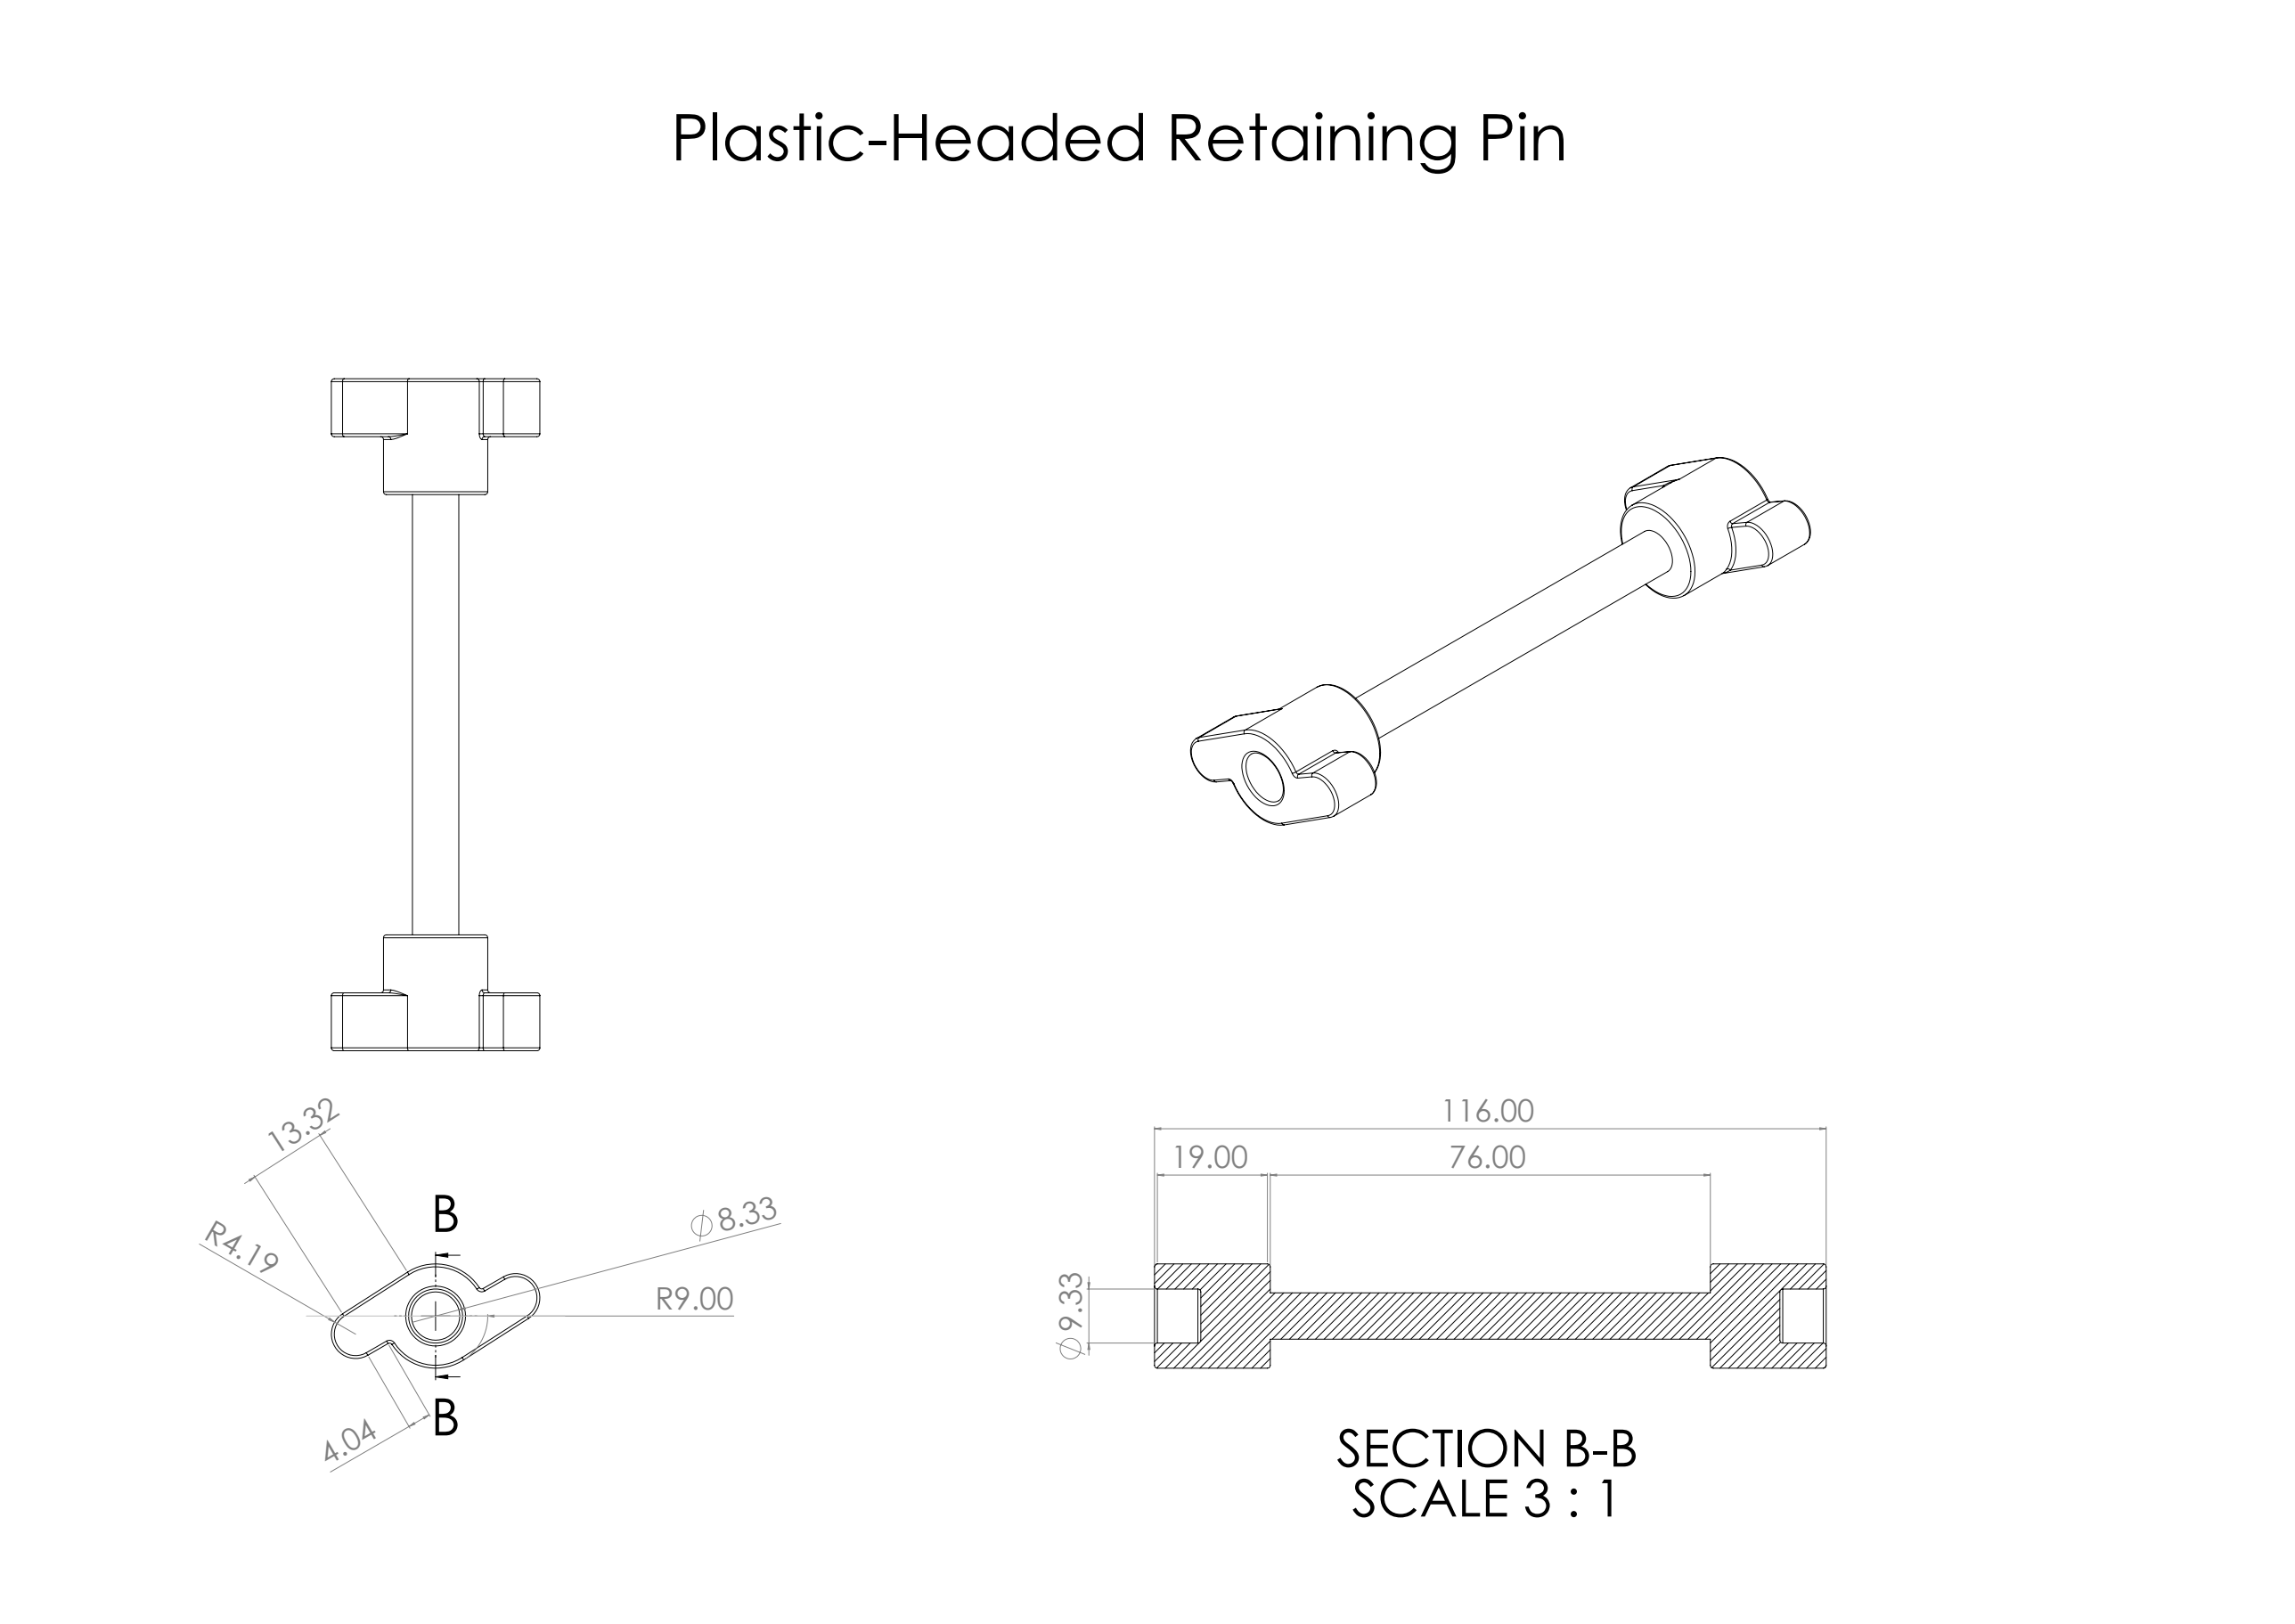
ISO-10303-21;
HEADER;
FILE_DESCRIPTION (('STEP AP214'),
    '1' );
FILE_NAME ('Plastic-Headed Retaining Pin.step',
    '2026-10-24T21:31:31',
    ( '' ),
    ( '' ),
    'SwSTEP 2.0',
    'SolidWorks 2025',
    '' );
FILE_SCHEMA (( 'AUTOMOTIVE_DESIGN' ));
ENDSEC;

DATA;
#1=AXIS2_PLACEMENT_3D ( 'NONE', #1022, #12813, #2258 ) ;
#8=EDGE_CURVE ( 'NONE', #12161, #11292, #4111, .T. ) ;
#15=ORIENTED_EDGE ( 'NONE', *, *, #6036, .T. ) ;
#28=FACE_OUTER_BOUND ( 'NONE', #3772, .T. ) ;
#31=CARTESIAN_POINT ( 'NONE',  ( -24.73111225919155132, -6.857688092579577344, -47.70917337021941762 ) ) ;
#34=ORIENTED_EDGE ( 'NONE', *, *, #2571, .T. ) ;
#45=CIRCLE ( 'NONE', #9384, 9.000000000000001776 ) ;
#48=CARTESIAN_POINT ( 'NONE',  ( -24.79038709231510040, -6.757381419356298657, 47.62582736825572738 ) ) ;
#51=ORIENTED_EDGE ( 'NONE', *, *, #11161, .F. ) ;
#53=VECTOR ( 'NONE', #9034, 1000.000000000000000 ) ;
#56=VERTEX_POINT ( 'NONE', #6360 ) ;
#60=VERTEX_POINT ( 'NONE', #14733 ) ;
#64=MECHANICAL_DESIGN_GEOMETRIC_PRESENTATION_REPRESENTATION('',(#7176),#14543);
#71=ORIENTED_EDGE ( 'NONE', *, *, #11240, .T. ) ;
#80=CIRCLE ( 'NONE', #11854, 0.5000000000000000000 ) ;
#83=CARTESIAN_POINT ( 'NONE',  ( -24.54250511040913096, 2.674312581063694516, -47.50000000000008527 ) ) ;
#90=DIRECTION ( 'NONE',  ( 0.000000000000000000, 0.000000000000000000, -1.000000000000000000 ) ) ;
#92=APPLICATION_CONTEXT ( 'automotive_design' ) ;
#93=CARTESIAN_POINT ( 'NONE',  ( -30.80945343098651890, -5.389243620311580329, -57.50000000000012079 ) ) ;
#103=( NAMED_UNIT ( * ) PLANE_ANGLE_UNIT ( ) SI_UNIT ( $, .RADIAN. ) );
#106=ORIENTED_EDGE ( 'NONE', *, *, #4616, .T. ) ;
#107=CARTESIAN_POINT ( 'NONE',  ( -9.038486528834313916, 1.949452350488303454, -47.50000000626571506 ) ) ;
#115=EDGE_LOOP ( 'NONE', ( #13949, #4522, #9265, #7527 ) ) ;
#119=CARTESIAN_POINT ( 'NONE',  ( -3.190546569013415379, 0.8906624217387615339, -57.50000000000012079 ) ) ;
#127=CARTESIAN_POINT ( 'NONE',  ( -25.21252699837112132, -6.998437922861948657, 48.50000000000011369 ) ) ;
#134=ORIENTED_EDGE ( 'NONE', *, *, #9339, .T. ) ;
#151=CARTESIAN_POINT ( 'NONE',  ( -22.13891797369473480, 5.141277655368648780, -48.38337049880507834 ) ) ;
#155=LINE ( 'NONE', #2612, #2752 ) ;
#160=DIRECTION ( 'NONE',  ( -0.000000000000000000, -0.000000000000000000, -1.000000000000000000 ) ) ;
#162=DIRECTION ( 'NONE',  ( 0.000000000000000000, 0.000000000000000000, 1.000000000000000000 ) ) ;
#164=CARTESIAN_POINT ( 'NONE',  ( -24.34296084301338681, 2.966536634491813818, 47.54128347412125066 ) ) ;
#165=EDGE_CURVE ( 'NONE', #11054, #3062, #11494, .T. ) ;
#169=AXIS2_PLACEMENT_3D ( 'NONE', #4841, #13010, #2308 ) ;
#170=VERTEX_POINT ( 'NONE', #13972 ) ;
#172=LINE ( 'NONE', #1320, #11742 ) ;
#175=CARTESIAN_POINT ( 'NONE',  ( -9.097850607046364502, 2.059891325575069043, -47.52616914649232172 ) ) ;
#193=TOROIDAL_SURFACE ( 'NONE', #8776, 5.165819364273509073, 0.5000000000000000000 ) ;
#198=CARTESIAN_POINT ( 'NONE',  ( -25.01741698508091005, -6.338425579613558014, 48.00000000000010658 ) ) ;
#202=ADVANCED_FACE ( 'NONE', ( #3509 ), #12825, .F. ) ;
#203=VECTOR ( 'NONE', #10665, 1000.000000000000000 ) ;
#210=CARTESIAN_POINT ( 'NONE',  ( 1.004339113574583608, 0.8906624217387615339, -48.00000000000012079 ) ) ;
#214=EDGE_CURVE ( 'NONE', #14442, #11277, #7315, .T. ) ;
#215=CIRCLE ( 'NONE', #445, 0.5000000000000000000 ) ;
#217=DIRECTION ( 'NONE',  ( -0.000000000000000000, 0.000000000000000000, 1.000000000000000000 ) ) ;
#219=DIRECTION ( 'NONE',  ( 0.8420378618367728718, 0.5394184268574404584, -0.000000000000000000 ) ) ;
#229=AXIS2_PLACEMENT_3D ( 'NONE', #14012, #3468, #10624 ) ;
#231=EDGE_LOOP ( 'NONE', ( #10918, #12061, #5408, #5048 ) ) ;
#241=CARTESIAN_POINT ( 'NONE',  ( -28.95977857253349796, -8.587818791446737876, 48.00000000000012079 ) ) ;
#244=CARTESIAN_POINT ( 'NONE',  ( -23.91311688008704905, 3.524160940036151324, 47.66502101098827637 ) ) ;
#250=CIRCLE ( 'NONE', #10335, 1.000000000000000888 ) ;
#253=CARTESIAN_POINT ( 'NONE',  ( -10.99067925302910176, -8.982598353005794678, -48.14374739243442747 ) ) ;
#267=FACE_OUTER_BOUND ( 'NONE', #14593, .T. ) ;
#269=ORIENTED_EDGE ( 'NONE', *, *, #14642, .F. ) ;
#274=CARTESIAN_POINT ( 'NONE',  ( -24.96483633670257873, -6.441926561070030033, 48.01692658285762150 ) ) ;
#282=AXIS2_PLACEMENT_3D ( 'NONE', #9055, #1887, #6818 ) ;
#284=EDGE_CURVE ( 'NONE', #12776, #11451, #5880, .T. ) ;
#290=CARTESIAN_POINT ( 'NONE',  ( -25.46282903980762669, -6.565599745187292946, 47.50000000000012079 ) ) ;
#296=ORIENTED_EDGE ( 'NONE', *, *, #1661, .T. ) ;
#298=VERTEX_POINT ( 'NONE', #5547 ) ;
#303=FACE_OUTER_BOUND ( 'NONE', #6423, .T. ) ;
#310=CIRCLE ( 'NONE', #8176, 4.665819364273509073 ) ;
#319=FACE_OUTER_BOUND ( 'NONE', #4555, .T. ) ;
#324=ORIENTED_EDGE ( 'NONE', *, *, #7653, .T. ) ;
#329=CARTESIAN_POINT ( 'NONE',  ( -9.191242442328487527, 2.249476921181321476, -48.36238429206942868 ) ) ;
#336=CIRCLE ( 'NONE', #6243, 3.694885682587998765 ) ;
#342=DIRECTION ( 'NONE',  ( 0.000000000000000000, 0.000000000000000000, 1.000000000000000000 ) ) ;
#345=DIRECTION ( 'NONE',  ( 0.000000000000000000, -0.000000000000000000, -1.000000000000000000 ) ) ;
#349=EDGE_CURVE ( 'NONE', #13079, #8396, #2395, .T. ) ;
#350=DIRECTION ( 'NONE',  ( -0.8656763553493062036, -0.5006040828730242698, -0.000000000000000000 ) ) ;
#353=ORIENTED_EDGE ( 'NONE', *, *, #9943, .F. ) ;
#355=VERTEX_POINT ( 'NONE', #12871 ) ;
#356=CARTESIAN_POINT ( 'NONE',  ( -25.46282903980762669, -6.565599745187292946, 48.00000000000012079 ) ) ;
#361=CARTESIAN_POINT ( 'NONE',  ( -32.80254285330622110, -2.278009980413880697, -48.50000000000012079 ) ) ;
#372=DIRECTION ( 'NONE',  ( 1.000000000000000000, 0.000000000000000000, 0.000000000000000000 ) ) ;
#373=ORIENTED_EDGE ( 'NONE', *, *, #13891, .T. ) ;
#375=ORIENTED_EDGE ( 'NONE', *, *, #2546, .T. ) ;
#376=DIRECTION ( 'NONE',  ( -0.000000000000000000, -0.000000000000000000, -1.000000000000000000 ) ) ;
#385=CARTESIAN_POINT ( 'NONE',  ( -24.57377864815406099, 2.621914368698142983, 47.92899112040971943 ) ) ;
#386=EDGE_CURVE ( 'NONE', #5046, #7147, #1076, .T. ) ;
#388=EDGE_CURVE ( 'NONE', #5785, #8918, #8303, .T. ) ;
#396=CARTESIAN_POINT ( 'NONE',  ( -10.31873516982594907, -8.289185193041582522, -47.74939190649462972 ) ) ;
#397=AXIS2_PLACEMENT_3D ( 'NONE', #6924, #8082, #15007 ) ;
#403=CARTESIAN_POINT ( 'NONE',  ( -8.729485970062036415, 2.417371407811747197, 48.19241902544784750 ) ) ;
#413=AXIS2_PLACEMENT_3D ( 'NONE', #11900, #10826, #1359 ) ;
#415=CARTESIAN_POINT ( 'NONE',  ( -25.21252699939434194, -6.998437923453657561, -48.43453164808065736 ) ) ;
#419=ADVANCED_BREP_SHAPE_REPRESENTATION ( '', ( #14292, #6315 ), #9517 ) ;
#426=AXIS2_PLACEMENT_3D ( 'NONE', #9506, #14202, #3798 ) ;
#429=DIRECTION ( 'NONE',  ( 0.000000000000000000, 0.000000000000000000, 1.000000000000000000 ) ) ;
#434=ORIENTED_EDGE ( 'NONE', *, *, #386, .T. ) ;
#443=ORIENTED_EDGE ( 'NONE', *, *, #5395, .T. ) ;
#444=CARTESIAN_POINT ( 'NONE',  ( -23.91237149244958360, 3.525053131390499139, 47.66527511103321046 ) ) ;
#445=AXIS2_PLACEMENT_3D ( 'NONE', #12775, #5776, #7923 ) ;
#451=AXIS2_PLACEMENT_3D ( 'NONE', #9024, #9337, #11476 ) ;
#452=CARTESIAN_POINT ( 'NONE',  ( -24.54316048551696028, -7.158540021523408292, 58.00000000000012079 ) ) ;
#455=DIRECTION ( 'NONE',  ( -0.5394184268574523378, 0.8420378618367652113, 0.000000000000000000 ) ) ;
#458=LINE ( 'NONE', #7761, #5187 ) ;
#459=DIRECTION ( 'NONE',  ( -0.5394184268574406804, 0.8420378618367728718, 0.000000000000000000 ) ) ;
#469=CARTESIAN_POINT ( 'NONE',  ( -9.657716696386627220, -7.466071317230740689, -47.54143911729025973 ) ) ;
#473=DIRECTION ( 'NONE',  ( -0.8420378618367644341, -0.5394184268574535590, -0.000000000000000000 ) ) ;
#478=CARTESIAN_POINT ( 'NONE',  ( -9.107478285483566083, 2.086796655788927701, 48.09696226170978406 ) ) ;
#485=EDGE_CURVE ( 'NONE', #14513, #11292, #5381, .T. ) ;
#486=AXIS2_PLACEMENT_3D ( 'NONE', #549, #8705, #618 ) ;
#487=EDGE_CURVE ( 'NONE', #14705, #9017, #2919, .T. ) ;
#490=VERTEX_POINT ( 'NONE', #4780 ) ;
#492=ORIENTED_EDGE ( 'NONE', *, *, #7012, .F. ) ;
#493=CARTESIAN_POINT ( 'NONE',  ( -25.24562193491511763, -6.954963132161501527, 48.23869654929341522 ) ) ;
#495=VECTOR ( 'NONE', #4431, 1000.000000000000000 ) ;
#498=ORIENTED_EDGE ( 'NONE', *, *, #9078, .F. ) ;
#499=PLANE ( 'NONE',  #14653 ) ;
#503=EDGE_CURVE ( 'NONE', #4611, #7961, #14234, .T. ) ;
#505=VERTEX_POINT ( 'NONE', #2771 ) ;
#509=ORIENTED_EDGE ( 'NONE', *, *, #3414, .F. ) ;
#511=ORIENTED_EDGE ( 'NONE', *, *, #11557, .T. ) ;
#516=DIRECTION ( 'NONE',  ( 0.000000000000000000, 0.000000000000000000, -1.000000000000000000 ) ) ;
#522=CIRCLE ( 'NONE', #13552, 0.5000000000000004441 ) ;
#528=DIRECTION ( 'NONE',  ( 1.000000000000000000, 0.000000000000000000, 0.000000000000000000 ) ) ;
#532=VECTOR ( 'NONE', #9239, 1000.000000000000000 ) ;
#545=AXIS2_PLACEMENT_3D ( 'NONE', #1167, #6104, #8339 ) ;
#546=ORIENTED_EDGE ( 'NONE', *, *, #487, .F. ) ;
#548=CIRCLE ( 'NONE', #9166, 0.5000000000000000000 ) ;
#549=CARTESIAN_POINT ( 'NONE',  ( -3.190546569013415379, 0.8906624217387615339, 48.50000000000012079 ) ) ;
#593=CARTESIAN_POINT ( 'NONE',  ( -9.657716696386627220, -7.466071317230740689, 47.54143911729025973 ) ) ;
#594=ORIENTED_EDGE ( 'NONE', *, *, #11102, .F. ) ;
#601=EDGE_LOOP ( 'NONE', ( #14385, #13165, #13920, #13167 ) ) ;
#603=ORIENTED_EDGE ( 'NONE', *, *, #12571, .F. ) ;
#616=ORIENTED_EDGE ( 'NONE', *, *, #4933, .T. ) ;
#618=DIRECTION ( 'NONE',  ( 1.000000000000000000, 0.000000000000000000, 0.000000000000000000 ) ) ;
#631=ORIENTED_EDGE ( 'NONE', *, *, #11253, .F. ) ;
#636=ORIENTED_EDGE ( 'NONE', *, *, #8900, .T. ) ;
#641=EDGE_CURVE ( 'NONE', #13513, #7657, #11510, .T. ) ;
#646=AXIS2_PLACEMENT_3D ( 'NONE', #2800, #14494, #8783 ) ;
#655=DIRECTION ( 'NONE',  ( 1.000000000000000000, 0.000000000000000000, 0.000000000000000000 ) ) ;
#663=EDGE_CURVE ( 'NONE', #4371, #14705, #1159, .T. ) ;
#664=DIRECTION ( 'NONE',  ( 1.000000000000000000, 0.000000000000000000, 0.000000000000000000 ) ) ;
#670=CARTESIAN_POINT ( 'NONE',  ( -32.80254285330626374, -2.278009980413908231, 48.50000000000012079 ) ) ;
#673=FACE_OUTER_BOUND ( 'NONE', #12478, .T. ) ;
#674=ORIENTED_EDGE ( 'NONE', *, *, #4052, .T. ) ;
#677=ORIENTED_EDGE ( 'NONE', *, *, #11895, .F. ) ;
#681=CARTESIAN_POINT ( 'NONE',  ( -24.66543232906180805, 3.122884019241207287, -48.02064173568555816 ) ) ;
#683=ORIENTED_EDGE ( 'NONE', *, *, #5858, .F. ) ;
#687=CARTESIAN_POINT ( 'NONE',  ( 0.000000000000000000, 0.000000000000000000, -38.00000000000012079 ) ) ;
#693=CARTESIAN_POINT ( 'NONE',  ( -16.99999999999998579, -2.249290599286303927, -57.50000000000012079 ) ) ;
#705=CARTESIAN_POINT ( 'NONE',  ( -24.55671735758753726, -7.137878559097176279, -48.23807154671105479 ) ) ;
#707=EDGE_CURVE ( 'NONE', #355, #7994, #45, .T. ) ;
#718=AXIS2_PLACEMENT_3D ( 'NONE', #2213, #10452, #821 ) ;
#727=EDGE_LOOP ( 'NONE', ( #10150, #492, #10188, #14509 ) ) ;
#730=FACE_OUTER_BOUND ( 'NONE', #5305, .T. ) ;
#744=CYLINDRICAL_SURFACE ( 'NONE', #11640, 0.4999999999999996669 ) ;
#746=AXIS2_PLACEMENT_3D ( 'NONE', #2112, #5754, #6809 ) ;
#748=DIRECTION ( 'NONE',  ( 0.5006040828730401460, -0.8656763553492970997, 0.000000000000000000 ) ) ;
#752=CARTESIAN_POINT ( 'NONE',  ( -21.58505662828840599, 4.908031226326156293, -57.50000000000012079 ) ) ;
#754=CIRCLE ( 'NONE', #12822, 0.4999999999999997224 ) ;
#763=LINE ( 'NONE', #1921, #4404 ) ;
#769=TOROIDAL_SURFACE ( 'NONE', #2002, 3.694885682587998765, 0.5000000000000000000 ) ;
#776=DIRECTION ( 'NONE',  ( 0.000000000000000000, 0.000000000000000000, -1.000000000000000000 ) ) ;
#779=AXIS2_PLACEMENT_3D ( 'NONE', #15041, #4571, #14877 ) ;
#781=AXIS2_PLACEMENT_3D ( 'NONE', #13323, #5092, #9797 ) ;
#785=CARTESIAN_POINT ( 'NONE',  ( -8.499999999999987566, -2.249290599286303927, -38.00000000000012079 ) ) ;
#789=CYLINDRICAL_SURFACE ( 'NONE', #12032, 4.194885682588113340 ) ;
#805=DIRECTION ( 'NONE',  ( 1.000000000000000000, 0.000000000000000000, 0.000000000000000000 ) ) ;
#821=DIRECTION ( 'NONE',  ( 1.000000000000000000, 0.000000000000000000, 0.000000000000000000 ) ) ;
#825=ORIENTED_EDGE ( 'NONE', *, *, #1492, .T. ) ;
#842=DIRECTION ( 'NONE',  ( -0.000000000000000000, -0.000000000000000000, -1.000000000000000000 ) ) ;
#851=ADVANCED_FACE ( 'NONE', ( #9652 ), #14341, .F. ) ;
#856=DIRECTION ( 'NONE',  ( 0.000000000000000000, -1.000000000000000000, 0.000000000000000000 ) ) ;
#859=FACE_OUTER_BOUND ( 'NONE', #13100, .T. ) ;
#864=VERTEX_POINT ( 'NONE', #12532 ) ;
#872=DIRECTION ( 'NONE',  ( 0.000000000000000000, 0.000000000000000000, -1.000000000000000000 ) ) ;
#877=DIRECTION ( 'NONE',  ( 1.000000000000000000, 0.000000000000000000, 0.000000000000000000 ) ) ;
#887=CARTESIAN_POINT ( 'NONE',  ( -16.99999999999998579, -2.249290599286303927, -58.00000000000012079 ) ) ;
#888=CIRCLE ( 'NONE', #9509, 0.4999999999999997780 ) ;
#890=CARTESIAN_POINT ( 'NONE',  ( -8.537170960192302260, 2.067018546614596719, -48.00000000000012079 ) ) ;
#892=AXIS2_PLACEMENT_3D ( 'NONE', #6524, #1690, #528 ) ;
#894=ORIENTED_EDGE ( 'NONE', *, *, #4866, .T. ) ;
#896=DIRECTION ( 'NONE',  ( 1.000000000000000000, 0.000000000000000000, 0.000000000000000000 ) ) ;
#901=EDGE_CURVE ( 'NONE', #298, #3805, #11869, .T. ) ;
#903=CARTESIAN_POINT ( 'NONE',  ( -7.499999999999985789, -2.249290599286303927, 47.50000000000012079 ) ) ;
#904=VECTOR ( 'NONE', #10762, 1000.000000000000114 ) ;
#912=CARTESIAN_POINT ( 'NONE',  ( -21.85476584171706449, 5.329050157244580532, -48.50000000000012079 ) ) ;
#915=EDGE_LOOP ( 'NONE', ( #9268, #4270, #12205, #3537 ) ) ;
#922=VERTEX_POINT ( 'NONE', #11287 ) ;
#933=CARTESIAN_POINT ( 'NONE',  ( -8.787473000605775297, 2.499856724880853864, -48.43453164808066447 ) ) ;
#934=CARTESIAN_POINT ( 'NONE',  ( -33.07225206673494711, -1.856991049495498425, -48.50000000000012079 ) ) ;
#936=DIRECTION ( 'NONE',  ( 0.8420378618367728718, 0.5394184268574404584, 0.000000000000000000 ) ) ;
#944=CARTESIAN_POINT ( 'NONE',  ( -28.70947653109703523, -9.020656969121422009, -57.50000000000012079 ) ) ;
#952=AXIS2_PLACEMENT_3D ( 'NONE', #10166, #3233, #14775 ) ;
#953=( BOUNDED_SURFACE ( )  B_SPLINE_SURFACE ( 3, 2, ( 
 ( #11003, #4136, #12769 ),
 ( #2218, #2299, #5613 ),
 ( #975, #5847, #11363 ),
 ( #7840, #12685, #2137 ),
 ( #3216, #9227, #15146 ),
 ( #15078, #3141, #6830 ),
 ( #14908, #3450, #10455 ),
 ( #8147, #10379, #10303 ) ),
 .UNSPECIFIED., .F., .F., .F. ) 
 B_SPLINE_SURFACE_WITH_KNOTS ( ( 4, 2, 2, 4 ),
 ( 3, 3 ),
 ( -6.505213034913026604E-19, 0.001129222206655588513, 0.002258444413311177894, 0.004516888826622356655 ),
 ( 0.000000000000000000, 1.000000000000000000 ),
 .UNSPECIFIED. ) 
 GEOMETRIC_REPRESENTATION_ITEM ( )  RATIONAL_B_SPLINE_SURFACE ( (
 ( 1.000000000000000000, 0.7071067811864926167, 1.000000000000000000),
 ( 1.000000000000000000, 0.7608707698419998611, 1.000000000000000000),
 ( 1.000000000000000000, 0.8047257278452493168, 1.000000000000000000),
 ( 1.000000000000000000, 0.8783509392183369568, 1.000000000000000000),
 ( 1.000000000000000000, 0.9081758943107525184, 1.000000000000000000),
 ( 1.000000000000000000, 0.9781389570701306546, 1.000000000000000000),
 ( 1.000000000000000000, 0.9996704379322433054, 1.000000000000000000),
 ( 1.000000000000000000, 1.000000000000000000, 1.000000000000000000) ) ) 
 REPRESENTATION_ITEM ( '' )  SURFACE ( )  );
#954=DIRECTION ( 'NONE',  ( 0.8420378618367644341, 0.5394184268574535590, 0.000000000000000000 ) ) ;
#956=CARTESIAN_POINT ( 'NONE',  ( 0.6601805061683232445, -1.030548743169294346, 57.50000000000012079 ) ) ;
#961=ORIENTED_EDGE ( 'NONE', *, *, #6671, .T. ) ;
#964=AXIS2_PLACEMENT_3D ( 'NONE', #11793, #936, #4486 ) ;
#968=ORIENTED_EDGE ( 'NONE', *, *, #5858, .T. ) ;
#971=FACE_OUTER_BOUND ( 'NONE', #5210, .T. ) ;
#974=EDGE_CURVE ( 'NONE', #11391, #10817, #14814, .T. ) ;
#975=CARTESIAN_POINT ( 'NONE',  ( -9.657039156986668260, -7.465117833064532249, 47.54128347411995037 ) ) ;
#981=VERTEX_POINT ( 'NONE', #6749 ) ;
#986=CYLINDRICAL_SURFACE ( 'NONE', #5207, 4.665819364273509073 ) ;
#988=ORIENTED_EDGE ( 'NONE', *, *, #12071, .F. ) ;
#990=VECTOR ( 'NONE', #350, 1000.000000000000000 ) ;
#994=DIRECTION ( 'NONE',  ( -0.000000000000000000, -0.000000000000000000, -1.000000000000000000 ) ) ;
#1006=ORIENTED_EDGE ( 'NONE', *, *, #15185, .F. ) ;
#1009=EDGE_LOOP ( 'NONE', ( #9822, #6669, #1334, #10838 ) ) ;
#1014=PLANE ( 'NONE',  #7092 ) ;
#1021=ORIENTED_EDGE ( 'NONE', *, *, #8257, .F. ) ;
#1022=CARTESIAN_POINT ( 'NONE',  ( -24.96222495693456978, -7.431276100536581275, -48.50000000000012079 ) ) ;
#1028=PLANE ( 'NONE',  #14565 ) ;
#1031=EDGE_CURVE ( 'NONE', #922, #3003, #2788, .T. ) ;
#1048=LINE ( 'NONE', #210, #4481 ) ;
#1050=CARTESIAN_POINT ( 'NONE',  ( 1.004339113574583608, 0.8906624217387615339, 48.00000000000012079 ) ) ;
#1055=AXIS2_PLACEMENT_3D ( 'NONE', #3787, #9729, #7919 ) ;
#1057=VECTOR ( 'NONE', #994, 1000.000000000000000 ) ;
#1069=VECTOR ( 'NONE', #4442, 1000.000000000000000 ) ;
#1070=EDGE_LOOP ( 'NONE', ( #1164, #3149 ) ) ;
#1076=LINE ( 'NONE', #3311, #11234 ) ;
#1081=DIRECTION ( 'NONE',  ( -0.000000000000000000, -0.000000000000000000, -1.000000000000000000 ) ) ;
#1097=ADVANCED_FACE ( 'NONE', ( #8307 ), #11826, .F. ) ;
#1106=DIRECTION ( 'NONE',  ( -0.000000000000000000, 1.000000000000000000, 0.000000000000000000 ) ) ;
#1108=DIRECTION ( 'NONE',  ( 1.000000000000000000, 0.000000000000000000, 0.000000000000000000 ) ) ;
#1122=DIRECTION ( 'NONE',  ( 1.000000000000000000, 0.000000000000000000, 0.000000000000000000 ) ) ;
#1124=EDGE_CURVE ( 'NONE', #11720, #12161, #8919, .T. ) ;
#1125=VERTEX_POINT ( 'NONE', #10604 ) ;
#1133=VECTOR ( 'NONE', #7599, 1000.000000000000000 ) ;
#1142=ORIENTED_EDGE ( 'NONE', *, *, #4718, .F. ) ;
#1152=AXIS2_PLACEMENT_3D ( 'NONE', #12756, #4427, #9132 ) ;
#1159=CIRCLE ( 'NONE', #5842, 0.5000000000000008882 ) ;
#1164=ORIENTED_EDGE ( 'NONE', *, *, #7456, .T. ) ;
#1167=CARTESIAN_POINT ( 'NONE',  ( -32.80254285330622110, -2.278009980413880697, 48.50000000000012079 ) ) ;
#1170=CIRCLE ( 'NONE', #6821, 9.500000000000001776 ) ;
#1172=FACE_OUTER_BOUND ( 'NONE', #2030, .T. ) ;
#1174=AXIS2_PLACEMENT_3D ( 'NONE', #11340, #12661, #954 ) ;
#1187=CARTESIAN_POINT ( 'NONE',  ( -8.842479278987921631, -7.118053859731281463, -48.00000000000012079 ) ) ;
#1197=CARTESIAN_POINT ( 'NONE',  ( -16.99999999999998579, -2.249290599286303927, 50.00000000000012079 ) ) ;
#1198=CARTESIAN_POINT ( 'NONE',  ( -25.46282903980763024, -6.565599745187293834, 48.00000000000012079 ) ) ;
#1204=DIRECTION ( 'NONE',  ( 0.5454721580263366398, -0.8381289428352246551, 4.385647630081457888E-16 ) ) ;
#1220=EDGE_LOOP ( 'NONE', ( #9030, #9222, #106, #3497 ) ) ;
#1223=CARTESIAN_POINT ( 'NONE',  ( -23.91237149244958360, 3.525053131390499139, -47.66527511103321046 ) ) ;
#1228=FACE_OUTER_BOUND ( 'NONE', #1806, .T. ) ;
#1238=ORIENTED_EDGE ( 'NONE', *, *, #9123, .F. ) ;
#1244=DIRECTION ( 'NONE',  ( 0.000000000000000000, 0.000000000000000000, 1.000000000000000000 ) ) ;
#1248=PLANE ( 'NONE',  #2409 ) ;
#1252=AXIS2_PLACEMENT_3D ( 'NONE', #11270, #13666, #13822 ) ;
#1253=EDGE_LOOP ( 'NONE', ( #1021, #5256, #6232, #324 ) ) ;
#1259=FACE_OUTER_BOUND ( 'NONE', #10043, .T. ) ;
#1268=CARTESIAN_POINT ( 'NONE',  ( -25.43628086306388525, -6.625164433253370788, 48.00000000000012079 ) ) ;
#1273=AXIS2_PLACEMENT_3D ( 'NONE', #8800, #13496, #6352 ) ;
#1282=AXIS2_PLACEMENT_3D ( 'NONE', #2665, #5347, #6422 ) ;
#1291=DIRECTION ( 'NONE',  ( 0.000000000000000000, 0.000000000000000000, -1.000000000000000000 ) ) ;
#1295=FACE_OUTER_BOUND ( 'NONE', #8669, .T. ) ;
#1304=CARTESIAN_POINT ( 'NONE',  ( -24.12409601409935078, -6.885803942510236197, -57.50000000000012079 ) ) ;
#1307=CARTESIAN_POINT ( 'NONE',  ( -30.80945343098651890, -5.389243620311580329, -48.00000000000012079 ) ) ;
#1309=EDGE_CURVE ( 'NONE', #12008, #14442, #8458, .T. ) ;
#1310=DIRECTION ( 'NONE',  ( -0.8656763553492639041, -0.5006040828730973224, 0.000000000000000000 ) ) ;
#1317=CARTESIAN_POINT ( 'NONE',  ( -3.190546569013415379, 0.8906624217387615339, 48.50000000000012079 ) ) ;
#1320=CARTESIAN_POINT ( 'NONE',  ( -28.70947653109703168, -9.020656969121420232, 48.00000000000012079 ) ) ;
#1326=EDGE_CURVE ( 'NONE', #7147, #298, #13221, .T. ) ;
#1328=EDGE_CURVE ( 'NONE', #505, #1125, #2947, .T. ) ;
#1334=ORIENTED_EDGE ( 'NONE', *, *, #12288, .T. ) ;
#1335=EDGE_CURVE ( 'NONE', #6376, #5507, #5755, .T. ) ;
#1337=FACE_OUTER_BOUND ( 'NONE', #5812, .T. ) ;
#1340=DIRECTION ( 'NONE',  ( 1.000000000000000000, 0.000000000000000000, 0.000000000000000000 ) ) ;
#1343=CARTESIAN_POINT ( 'NONE',  ( -8.537170960192327129, 2.067018546614582508, 57.50000000000012079 ) ) ;
#1353=PRODUCT_DEFINITION_CONTEXT ( 'detailed design', #5158, 'design' ) ;
#1357=ORIENTED_EDGE ( 'NONE', *, *, #5945, .T. ) ;
#1359=DIRECTION ( 'NONE',  ( 1.000000000000000000, 0.000000000000000000, 0.000000000000000000 ) ) ;
#1366=LINE ( 'NONE', #2596, #12722 ) ;
#1368=ORIENTED_EDGE ( 'NONE', *, *, #8899, .T. ) ;
#1375=VERTEX_POINT ( 'NONE', #4186 ) ;
#1388=DIRECTION ( 'NONE',  ( -0.4543483311474630915, 0.8908241094534405935, -0.000000000000000000 ) ) ;
#1390=CARTESIAN_POINT ( 'NONE',  ( -24.54301448188264700, 2.673459138797629198, 47.50000001881890910 ) ) ;
#1393=CIRCLE ( 'NONE', #3357, 9.000000000000001776 ) ;
#1395=AXIS2_PLACEMENT_3D ( 'NONE', #2267, #15123, #11570 ) ;
#1399=CARTESIAN_POINT ( 'NONE',  ( -9.209612907684750382, 2.258800220783480750, -47.62582736825572738 ) ) ;
#1402=DIRECTION ( 'NONE',  ( 1.000000000000000000, 0.000000000000000000, 0.000000000000000000 ) ) ;
#1409=AXIS2_PLACEMENT_3D ( 'NONE', #11979, #4986, #10916 ) ;
#1421=CARTESIAN_POINT ( 'NONE',  ( -24.90214939295363550, -6.558472524147630267, 47.52616914649232172 ) ) ;
#1437=CIRCLE ( 'NONE', #6552, 0.5000000000000004441 ) ;
#1450=ORIENTED_EDGE ( 'NONE', *, *, #5868, .T. ) ;
#1453=ORIENTED_EDGE ( 'NONE', *, *, #4286, .F. ) ;
#1454=CARTESIAN_POINT ( 'NONE',  ( -16.99999999999998579, -2.249290599286303927, -47.50000000000012079 ) ) ;
#1455=CARTESIAN_POINT ( 'NONE',  ( -11.05444845021228595, -9.014367880605227867, 48.04486892757390848 ) ) ;
#1458=CARTESIAN_POINT ( 'NONE',  ( -3.285520523750506516, 5.681530634152946568, 48.00000000000012079 ) ) ;
#1462=( BOUNDED_SURFACE ( )  B_SPLINE_SURFACE ( 3, 2, ( 
 ( #5640, #10330, #9182 ),
 ( #13867, #8020, #12719 ),
 ( #5726, #9253, #13947 ),
 ( #8099, #12800, #14104 ),
 ( #2402, #10482, #11935 ),
 ( #11708, #253, #13104 ),
 ( #10566, #3556, #4711 ),
 ( #9573, #2479, #10713 ) ),
 .UNSPECIFIED., .F., .F., .F. ) 
 B_SPLINE_SURFACE_WITH_KNOTS ( ( 4, 2, 2, 4 ),
 ( 3, 3 ),
 ( -6.505213034913026604E-19, 0.001129222206655588513, 0.002258444413311177894, 0.004516888826622356655 ),
 ( 0.000000000000000000, 1.000000000000000000 ),
 .UNSPECIFIED. ) 
 GEOMETRIC_REPRESENTATION_ITEM ( )  RATIONAL_B_SPLINE_SURFACE ( (
 ( 1.000000000000000000, 0.7071067811864926167, 1.000000000000000000),
 ( 1.000000000000000000, 0.7608707698419998611, 1.000000000000000000),
 ( 1.000000000000000000, 0.8047257278452493168, 1.000000000000000000),
 ( 1.000000000000000000, 0.8783509392183369568, 1.000000000000000000),
 ( 1.000000000000000000, 0.9081758943107525184, 1.000000000000000000),
 ( 1.000000000000000000, 0.9781389570701306546, 1.000000000000000000),
 ( 1.000000000000000000, 0.9996704379322433054, 1.000000000000000000),
 ( 1.000000000000000000, 1.000000000000000000, 1.000000000000000000) ) ) 
 REPRESENTATION_ITEM ( '' )  SURFACE ( )  );
#1468=CARTESIAN_POINT ( 'NONE',  ( -0.9277479332649583021, -2.641590149077306826, -48.00000000000012079 ) ) ;
#1469=ORIENTED_EDGE ( 'NONE', *, *, #9614, .T. ) ;
#1473=AXIS2_PLACEMENT_3D ( 'NONE', #2874, #6349, #7729 ) ;
#1484=CARTESIAN_POINT ( 'NONE',  ( -25.01741698508091005, -6.338425579613558014, 47.50000000000012079 ) ) ;
#1485=CIRCLE ( 'NONE', #9354, 0.5000000000000001110 ) ;
#1488=CARTESIAN_POINT ( 'NONE',  ( -9.263396839842437558, 2.349907881949450772, 47.70033363922482295 ) ) ;
#1492=EDGE_CURVE ( 'NONE', #4595, #14705, #4581, .T. ) ;
#1507=CARTESIAN_POINT ( 'NONE',  ( -25.34493114703935035, -6.799303420495464323, 48.05421924268924272 ) ) ;
#1515=CARTESIAN_POINT ( 'NONE',  ( -32.80254285330626374, -2.278009980413909563, 48.00000000000012079 ) ) ;
#1521=AXIS2_PLACEMENT_3D ( 'NONE', #2798, #342, #6267 ) ;
#1531=EDGE_LOOP ( 'NONE', ( #3137, #10096, #134, #7878 ) ) ;
#1543=CARTESIAN_POINT ( 'NONE',  ( -25.49999999999998934, -2.249290599286304815, -38.50000000000012790 ) ) ;
#1544=DIRECTION ( 'NONE',  ( -0.000000000000000000, 0.000000000000000000, 1.000000000000000000 ) ) ;
#1553=ORIENTED_EDGE ( 'NONE', *, *, #485, .T. ) ;
#1564=DIRECTION ( 'NONE',  ( -0.000000000000000000, -0.000000000000000000, 1.000000000000000000 ) ) ;
#1566=EDGE_CURVE ( 'NONE', #2463, #8222, #8929, .T. ) ;
#1568=CARTESIAN_POINT ( 'NONE',  ( -9.191242442328487527, 2.249476921181321476, 48.36238429206942868 ) ) ;
#1579=EDGE_CURVE ( 'NONE', #7961, #60, #5669, .T. ) ;
#1588=DIRECTION ( 'NONE',  ( 0.000000000000000000, 0.000000000000000000, -1.000000000000000000 ) ) ;
#1605=CARTESIAN_POINT ( 'NONE',  ( -8.499999999999987566, -2.249290599286303927, 38.00000000000012079 ) ) ;
#1606=CARTESIAN_POINT ( 'NONE',  ( -32.80254285330622821, -2.278009980413885582, -58.00000000000012079 ) ) ;
#1613=DIRECTION ( 'NONE',  ( 1.000000000000000000, -2.602085213965208275E-15, 0.000000000000000000 ) ) ;
#1619=EDGE_CURVE ( 'NONE', #10926, #10853, #8787, .T. ) ;
#1620=DIRECTION ( 'NONE',  ( 1.000000000000000000, 0.000000000000000000, 0.000000000000000000 ) ) ;
#1621=ADVANCED_FACE ( 'NONE', ( #4560 ), #6714, .T. ) ;
#1625=CARTESIAN_POINT ( 'NONE',  ( -11.45041300328984413, -9.336677115435668028, -48.21133583021728697 ) ) ;
#1626=AXIS2_PLACEMENT_3D ( 'NONE', #9334, #2248, #15108 ) ;
#1630=DIRECTION ( 'NONE',  ( 1.000000000000000000, 0.000000000000000000, 0.000000000000000000 ) ) ;
#1634=CARTESIAN_POINT ( 'NONE',  ( -9.198099351547387670, 2.262399358110477543, 48.50000000000012079 ) ) ;
#1637=CARTESIAN_POINT ( 'NONE',  ( -12.41494337171168283, -9.406612424898836977, -57.50000000000012079 ) ) ;
#1640=VECTOR ( 'NONE', #3870, 1000.000000000000000 ) ;
#1643=ADVANCED_FACE ( 'NONE', ( #15110 ), #1014, .F. ) ;
#1661=EDGE_CURVE ( 'NONE', #11281, #5785, #1667, .T. ) ;
#1662=ADVANCED_FACE ( 'NONE', ( #3174 ), #11641, .T. ) ;
#1663=CARTESIAN_POINT ( 'NONE',  ( -16.99999999999998579, -2.249290599286303927, -50.00000000000012079 ) ) ;
#1667=CIRCLE ( 'NONE', #9049, 8.500000000000000000 ) ;
#1676=AXIS2_PLACEMENT_3D ( 'NONE', #10243, #7634, #6541 ) ;
#1677=ORIENTED_EDGE ( 'NONE', *, *, #13730, .F. ) ;
#1687=CARTESIAN_POINT ( 'NONE',  ( -16.99999999999998579, -2.249290599286303927, 47.50000000000012079 ) ) ;
#1690=DIRECTION ( 'NONE',  ( 0.000000000000000000, -0.000000000000000000, -1.000000000000000000 ) ) ;
#1708=VERTEX_POINT ( 'NONE', #934 ) ;
#1712=ORIENTED_EDGE ( 'NONE', *, *, #14627, .F. ) ;
#1714=CARTESIAN_POINT ( 'NONE',  ( -8.982583014919022446, 1.839844381040865118, 47.50000000000012079 ) ) ;
#1723=DIRECTION ( 'NONE',  ( 0.8420378618367644341, 0.5394184268574535590, -0.000000000000000000 ) ) ;
#1729=DIRECTION ( 'NONE',  ( -0.5394184268574414576, 0.8420378618367722057, 0.000000000000000000 ) ) ;
#1730=ORIENTED_EDGE ( 'NONE', *, *, #9732, .T. ) ;
#1731=CARTESIAN_POINT ( 'NONE',  ( -33.07225206673494711, -1.856991049495498425, -57.50000000000012079 ) ) ;
#1735=ORIENTED_EDGE ( 'NONE', *, *, #8857, .F. ) ;
#1737=CIRCLE ( 'NONE', #3474, 4.194885682587998765 ) ;
#1740=ORIENTED_EDGE ( 'NONE', *, *, #7059, .T. ) ;
#1741=VERTEX_POINT ( 'NONE', #2017 ) ;
#1742=CARTESIAN_POINT ( 'NONE',  ( -24.34228330361342785, 2.967490118658024034, 47.54143911729025973 ) ) ;
#1748=DIRECTION ( 'NONE',  ( -0.5006040828730989878, 0.8656763553492631269, 0.000000000000000000 ) ) ;
#1749=ORIENTED_EDGE ( 'NONE', *, *, #13506, .F. ) ;
#1753=CIRCLE ( 'NONE', #2253, 4.194885682587998765 ) ;
#1754=VECTOR ( 'NONE', #9423, 1000.000000000000000 ) ;
#1761=ORIENTED_EDGE ( 'NONE', *, *, #12757, .T. ) ;
#1767=DIRECTION ( 'NONE',  ( -0.000000000000000000, 0.000000000000000000, 1.000000000000000000 ) ) ;
#1769=DIRECTION ( 'NONE',  ( 0.000000000000000000, 0.000000000000000000, -1.000000000000000000 ) ) ;
#1770=EDGE_LOOP ( 'NONE', ( #3230, #8616, #5674, #9924 ) ) ;
#1784=ORIENTED_EDGE ( 'NONE', *, *, #10860, .F. ) ;
#1789=EDGE_CURVE ( 'NONE', #6376, #7757, #8319, .T. ) ;
#1794=AXIS2_PLACEMENT_3D ( 'NONE', #1663, #5129, #10911 ) ;
#1796=CARTESIAN_POINT ( 'NONE',  ( -8.779641963837230279, 13.70511383897430058, 48.00000000000012079 ) ) ;
#1797=ADVANCED_FACE ( 'NONE', ( #11713 ), #5355, .T. ) ;
#1798=CARTESIAN_POINT ( 'NONE',  ( -25.24934951899391322, -6.946659123520668722, -48.24789848114230040 ) ) ;
#1802=CIRCLE ( 'NONE', #4246, 0.5000000000000000000 ) ;
#1805=LINE ( 'NONE', #11184, #8891 ) ;
#1806=EDGE_LOOP ( 'NONE', ( #9387, #9780, #1784, #11783 ) ) ;
#1808=CARTESIAN_POINT ( 'NONE',  ( -8.787473001628837821, 2.499856724289235554, -58.00000000000012079 ) ) ;
#1816=ORIENTED_EDGE ( 'NONE', *, *, #13193, .F. ) ;
#1823=EDGE_CURVE ( 'NONE', #8849, #1741, #9036, .T. ) ;
#1831=DIRECTION ( 'NONE',  ( 0.000000000000000000, 0.000000000000000000, -1.000000000000000000 ) ) ;
#1837=ORIENTED_EDGE ( 'NONE', *, *, #7544, .T. ) ;
#1840=CARTESIAN_POINT ( 'NONE',  ( -23.87164973098472487, 3.842474614898954144, -48.12459668492483189 ) ) ;
#1854=AXIS2_PLACEMENT_3D ( 'NONE', #11866, #11937, #6259 ) ;
#1856=EDGE_LOOP ( 'NONE', ( #14590, #12513, #2901, #14475, #594, #2880, #7996, #8140, #13898, #988 ) ) ;
#1868=ADVANCED_FACE ( 'NONE', ( #28 ), #1248, .F. ) ;
#1871=FACE_BOUND ( 'NONE', #1070, .T. ) ;
#1877=CIRCLE ( 'NONE', #8034, 0.5000000000000004441 ) ;
#1887=DIRECTION ( 'NONE',  ( -0.000000000000000000, -0.000000000000000000, 1.000000000000000000 ) ) ;
#1897=DIRECTION ( 'NONE',  ( 0.8656763553493057595, 0.5006040828730249359, 0.000000000000000000 ) ) ;
#1915=CARTESIAN_POINT ( 'NONE',  ( -30.80945343098651890, -5.389243620311580329, -48.50000000000012079 ) ) ;
#1916=CARTESIAN_POINT ( 'NONE',  ( -21.85476584171706449, 5.329050157244581420, -48.50000000000012079 ) ) ;
#1921=CARTESIAN_POINT ( 'NONE',  ( -12.33418063572647938, -2.249290599286303927, -50.00000000000012079 ) ) ;
#1922=CARTESIAN_POINT ( 'NONE',  ( -32.80254285330622110, -2.278009980413881141, -58.00000000000012079 ) ) ;
#1928=EDGE_CURVE ( 'NONE', #7657, #12792, #11487, .T. ) ;
#1936=DIRECTION ( 'NONE',  ( 0.5394184268574535590, -0.8420378618367644341, 0.000000000000000000 ) ) ;
#1939=CARTESIAN_POINT ( 'NONE',  ( -24.89252171451660445, -6.585377854361484040, -48.09696226170979827 ) ) ;
#1940=EDGE_LOOP ( 'NONE', ( #13963, #5839, #12386, #9978 ) ) ;
#1943=ORIENTED_EDGE ( 'NONE', *, *, #9943, .T. ) ;
#1952=ADVANCED_FACE ( 'NONE', ( #2039 ), #14463, .T. ) ;
#1957=CARTESIAN_POINT ( 'NONE',  ( -16.99999999999998579, -2.249290599286303927, -50.50000000000012079 ) ) ;
#1961=VERTEX_POINT ( 'NONE', #13894 ) ;
#1963=ORIENTED_EDGE ( 'NONE', *, *, #10035, .T. ) ;
#1970=PLANE ( 'NONE',  #11844 ) ;
#1979=ORIENTED_EDGE ( 'NONE', *, *, #6666, .F. ) ;
#1980=TOROIDAL_SURFACE ( 'NONE', #12070, 8.500000000000000000, 0.5000000000000000000 ) ;
#1985=ORIENTED_EDGE ( 'NONE', *, *, #12699, .T. ) ;
#1989=CARTESIAN_POINT ( 'NONE',  ( -24.91612020358099855, 2.875255380930533455, -48.00000000000010658 ) ) ;
#1995=DIRECTION ( 'NONE',  ( 1.000000000000000000, 0.000000000000000000, 0.000000000000000000 ) ) ;
#2000=CYLINDRICAL_SURFACE ( 'NONE', #1676, 0.5000000000000001110 ) ;
#2002=AXIS2_PLACEMENT_3D ( 'NONE', #5472, #5783, #13619 ) ;
#2006=( NAMED_UNIT ( * ) SI_UNIT ( $, .STERADIAN. ) SOLID_ANGLE_UNIT ( ) );
#2015=AXIS2_PLACEMENT_3D ( 'NONE', #4791, #3637, #10483 ) ;
#2017=CARTESIAN_POINT ( 'NONE',  ( 0.5043391135745837195, 0.8906624217387615339, -58.00000000000012079 ) ) ;
#2021=PLANE ( 'NONE',  #6174 ) ;
#2024=EDGE_LOOP ( 'NONE', ( #12450, #9299, #2404, #8022 ) ) ;
#2030=EDGE_LOOP ( 'NONE', ( #2808, #10539, #4606, #9460 ) ) ;
#2037=EDGE_CURVE ( 'NONE', #9017, #8990, #9439, .T. ) ;
#2039=FACE_OUTER_BOUND ( 'NONE', #12782, .T. ) ;
#2057=DIRECTION ( 'NONE',  ( 0.000000000000000000, 0.000000000000000000, -1.000000000000000000 ) ) ;
#2058=EDGE_CURVE ( 'NONE', #5785, #11281, #11021, .T. ) ;
#2069=ORIENTED_EDGE ( 'NONE', *, *, #8884, .T. ) ;
#2074=LINE ( 'NONE', #12546, #8885 ) ;
#2091=CARTESIAN_POINT ( 'NONE',  ( -9.456839514482959785, 2.659958822950722279, -48.50000000000011369 ) ) ;
#2092=CARTESIAN_POINT ( 'NONE',  ( -16.99999999999998579, -2.249290599286303927, 38.00000000000012079 ) ) ;
#2094=CARTESIAN_POINT ( 'NONE',  ( 0.5043391135745837195, 0.8906624217387615339, 57.50000000000012079 ) ) ;
#2100=ORIENTED_EDGE ( 'NONE', *, *, #7921, .T. ) ;
#2102=CYLINDRICAL_SURFACE ( 'NONE', #779, 4.194885682587998765 ) ;
#2105=VERTEX_POINT ( 'NONE', #10434 ) ;
#2108=CARTESIAN_POINT ( 'NONE',  ( -7.499999999999985789, -2.249290599286303927, -47.50000000000012079 ) ) ;
#2109=AXIS2_PLACEMENT_3D ( 'NONE', #1317, #8179, #5879 ) ;
#2112=CARTESIAN_POINT ( 'NONE',  ( -22.16581936427349575, -2.249290599286303483, 57.50000000000012079 ) ) ;
#2114=CARTESIAN_POINT ( 'NONE',  ( -25.21252699837112132, -6.998437922861944216, -48.36782213136056896 ) ) ;
#2125=ADVANCED_FACE ( 'NONE', ( #11576 ), #11734, .F. ) ;
#2130=DIRECTION ( 'NONE',  ( 0.000000000000000000, 0.000000000000000000, -1.000000000000000000 ) ) ;
#2137=CARTESIAN_POINT ( 'NONE',  ( -9.855956283963589470, -8.104443761338727015, 48.08251050686958905 ) ) ;
#2138=ORIENTED_EDGE ( 'NONE', *, *, #11839, .F. ) ;
#2141=ORIENTED_EDGE ( 'NONE', *, *, #2037, .T. ) ;
#2147=CARTESIAN_POINT ( 'NONE',  ( -23.68178719075091365, 3.790042057515504048, -47.74919337097016836 ) ) ;
#2152=DIRECTION ( 'NONE',  ( 0.000000000000000000, 0.000000000000000000, -1.000000000000000000 ) ) ;
#2160=CARTESIAN_POINT ( 'NONE',  ( -25.46282903980762669, -6.565599745187292946, -47.50000000000012079 ) ) ;
#2163=ORIENTED_EDGE ( 'NONE', *, *, #1566, .T. ) ;
#2166=AXIS2_PLACEMENT_3D ( 'NONE', #7072, #3298, #8152 ) ;
#2171=AXIS2_PLACEMENT_3D ( 'NONE', #6969, #7197, #1108 ) ;
#2173=CARTESIAN_POINT ( 'NONE',  ( -16.99999999999998579, -2.249290599286303927, -38.50000000000012790 ) ) ;
#2175=ADVANCED_FACE ( 'NONE', ( #4579 ), #8075, .F. ) ;
#2187=CARTESIAN_POINT ( 'NONE',  ( -32.80254285330622110, -2.278009980413880697, 48.00000000000012079 ) ) ;
#2196=CARTESIAN_POINT ( 'NONE',  ( -30.80945343098651890, -5.389243620311580329, 48.00000000000012079 ) ) ;
#2204=VECTOR ( 'NONE', #4280, 1000.000000000000000 ) ;
#2206=AXIS2_PLACEMENT_3D ( 'NONE', #13645, #14797, #3100 ) ;
#2207=ORIENTED_EDGE ( 'NONE', *, *, #11253, .T. ) ;
#2213=CARTESIAN_POINT ( 'NONE',  ( -3.190546569013415379, 0.8906624217387615339, -57.50000000000012079 ) ) ;
#2218=CARTESIAN_POINT ( 'NONE',  ( -9.456985518117400957, -7.172040337370347629, 47.50000001881890910 ) ) ;
#2221=VERTEX_POINT ( 'NONE', #14362 ) ;
#2225=AXIS2_PLACEMENT_3D ( 'NONE', #12713, #12477, #3242 ) ;
#2229=CARTESIAN_POINT ( 'NONE',  ( 0.9298897195970434737, -1.451567674087680837, -48.50000000000012079 ) ) ;
#2239=AXIS2_PLACEMENT_3D ( 'NONE', #8972, #14979, #9137 ) ;
#2248=DIRECTION ( 'NONE',  ( -0.000000000000000000, -0.000000000000000000, 1.000000000000000000 ) ) ;
#2250=AXIS2_PLACEMENT_3D ( 'NONE', #13282, #11115, #4974 ) ;
#2253=AXIS2_PLACEMENT_3D ( 'NONE', #4361, #3208, #664 ) ;
#2254=DIRECTION ( 'NONE',  ( -0.8420378618367735379, -0.5394184268574396812, 9.357418084440779321E-16 ) ) ;
#2258=DIRECTION ( 'NONE',  ( 1.000000000000000000, -1.214306433183763862E-14, 0.000000000000000000 ) ) ;
#2264=ORIENTED_EDGE ( 'NONE', *, *, #8967, .F. ) ;
#2266=CARTESIAN_POINT ( 'NONE',  ( -28.95977857253349796, -8.587818791446737876, 48.50000000000012079 ) ) ;
#2267=CARTESIAN_POINT ( 'NONE',  ( -3.535822565187055400, 6.114368811827579187, -57.50000000000012079 ) ) ;
#2274=CARTESIAN_POINT ( 'NONE',  ( -16.99999999999998579, -2.249290599286303927, 57.50000000000012079 ) ) ;
#2277=CARTESIAN_POINT ( 'NONE',  ( -25.46282903980762669, -6.565599745187292946, -48.00000000000012079 ) ) ;
#2284=FACE_OUTER_BOUND ( 'NONE', #1531, .T. ) ;
#2286=DIRECTION ( 'NONE',  ( 0.000000000000000000, -0.000000000000000000, -1.000000000000000000 ) ) ;
#2288=VERTEX_POINT ( 'NONE', #5788 ) ;
#2292=EDGE_CURVE ( 'NONE', #490, #10969, #9562, .T. ) ;
#2299=CARTESIAN_POINT ( 'NONE',  ( -9.426221351845022411, -7.120495567271055037, 47.92899112040987575 ) ) ;
#2308=DIRECTION ( 'NONE',  ( 1.000000000000000000, 0.000000000000000000, 0.000000000000000000 ) ) ;
#2319=ORIENTED_EDGE ( 'NONE', *, *, #3670, .F. ) ;
#2332=CARTESIAN_POINT ( 'NONE',  ( 0.9298897195970434737, -1.451567674087680837, 48.00000000000012079 ) ) ;
#2334=CARTESIAN_POINT ( 'NONE',  ( -24.89835624542414649, -6.565460432723037698, -47.52815511422343775 ) ) ;
#2353=ORIENTED_EDGE ( 'NONE', *, *, #4906, .T. ) ;
#2359=ORIENTED_EDGE ( 'NONE', *, *, #13889, .T. ) ;
#2364=AXIS2_PLACEMENT_3D ( 'NONE', #9489, #11788, #3706 ) ;
#2369=CARTESIAN_POINT ( 'NONE',  ( -24.54316048551696028, -7.158540021523408292, 57.50000000000012079 ) ) ;
#2371=LINE ( 'NONE', #4828, #9294 ) ;
#2373=VERTEX_POINT ( 'NONE', #10703 ) ;
#2375=DIRECTION ( 'NONE',  ( -0.000000000000000000, 0.000000000000000000, 1.000000000000000000 ) ) ;
#2383=AXIS2_PLACEMENT_3D ( 'NONE', #1454, #516, #14670 ) ;
#2387=ORIENTED_EDGE ( 'NONE', *, *, #11240, .F. ) ;
#2388=CARTESIAN_POINT ( 'NONE',  ( -25.49999999999998934, -2.249290599286303038, 38.50000000000012790 ) ) ;
#2389=DIRECTION ( 'NONE',  ( -0.5394184268574520047, 0.8420378618367654333, 0.000000000000000000 ) ) ;
#2391=DIRECTION ( 'NONE',  ( 1.000000000000000000, 0.000000000000000000, 0.000000000000000000 ) ) ;
#2393=ORIENTED_EDGE ( 'NONE', *, *, #4782, .T. ) ;
#2395=CIRCLE ( 'NONE', #2649, 8.500000000000000000 ) ;
#2402=CARTESIAN_POINT ( 'NONE',  ( -10.12835026901530178, -8.341055813471566438, -48.12459668492476084 ) ) ;
#2404=ORIENTED_EDGE ( 'NONE', *, *, #9772, .T. ) ;
#2409=AXIS2_PLACEMENT_3D ( 'NONE', #14187, #11940, #1402 ) ;
#2411=DIRECTION ( 'NONE',  ( 0.000000000000000000, 0.000000000000000000, 1.000000000000000000 ) ) ;
#2413=DIRECTION ( 'NONE',  ( 0.000000000000000000, -1.000000000000000000, 0.000000000000000000 ) ) ;
#2416=CIRCLE ( 'NONE', #9798, 0.5000000000000004441 ) ;
#2418=B_SPLINE_CURVE_WITH_KNOTS ( 'NONE', 3,
 ( #4851, #9560, #4781, #14244, #8400, #10781, #7160, #10625, #9476, #11775 ),
 .UNSPECIFIED., .F., .F.,
 ( 4, 2, 2, 2, 4 ),
 ( 0.000000000000000000, 0.0003835113287520873016, 0.0007670226575041746032, 0.001150533986256262013, 0.001534045315008349206 ),
 .UNSPECIFIED. ) ;
#2430=EDGE_CURVE ( 'NONE', #13978, #7020, #2418, .T. ) ;
#2437=ORIENTED_EDGE ( 'NONE', *, *, #1579, .T. ) ;
#2440=CARTESIAN_POINT ( 'NONE',  ( -0.9277479332649583021, -2.641590149077306826, -48.50000000000012079 ) ) ;
#2447=CYLINDRICAL_SURFACE ( 'NONE', #10266, 4.194885682587998765 ) ;
#2463=VERTEX_POINT ( 'NONE', #13163 ) ;
#2468=EDGE_CURVE ( 'NONE', #6074, #7994, #6913, .T. ) ;
#2470=FACE_OUTER_BOUND ( 'NONE', #8824, .T. ) ;
#2478=EDGE_CURVE ( 'NONE', #7490, #5809, #14168, .T. ) ;
#2479=CARTESIAN_POINT ( 'NONE',  ( -12.14523415828302078, -9.827631355817260328, -48.50000000000012079 ) ) ;
#2480=DIRECTION ( 'NONE',  ( -0.000000000000000000, 0.000000000000000000, -1.000000000000000000 ) ) ;
#2483=DIRECTION ( 'NONE',  ( 0.000000000000000000, 0.000000000000000000, -1.000000000000000000 ) ) ;
#2484=DIRECTION ( 'NONE',  ( 0.5006040828730989878, -0.8656763553492631269, 0.000000000000000000 ) ) ;
#2494=ORIENTED_EDGE ( 'NONE', *, *, #3193, .F. ) ;
#2496=ORIENTED_EDGE ( 'NONE', *, *, #2920, .F. ) ;
#2499=AXIS2_PLACEMENT_3D ( 'NONE', #14059, #1204, #14138 ) ;
#2500=CYLINDRICAL_SURFACE ( 'NONE', #12094, 0.5000000000000004441 ) ;
#2503=EDGE_CURVE ( 'NONE', #8531, #8396, #2984, .T. ) ;
#2513=ORIENTED_EDGE ( 'NONE', *, *, #13184, .F. ) ;
#2514=DIRECTION ( 'NONE',  ( 0.000000000000000000, 0.000000000000000000, -1.000000000000000000 ) ) ;
#2528=LINE ( 'NONE', #7217, #8314 ) ;
#2537=AXIS2_PLACEMENT_3D ( 'NONE', #2266, #8277, #6963 ) ;
#2538=EDGE_LOOP ( 'NONE', ( #7579, #9998, #4706, #1142 ) ) ;
#2539=AXIS2_PLACEMENT_3D ( 'NONE', #13607, #14906, #3214 ) ;
#2540=CARTESIAN_POINT ( 'NONE',  ( -21.99701278316016584, 5.237925250804929433, -48.44214661496815211 ) ) ;
#2543=CIRCLE ( 'NONE', #5989, 0.5000000000000004441 ) ;
#2546=EDGE_CURVE ( 'NONE', #11391, #7994, #3838, .T. ) ;
#2558=DIRECTION ( 'NONE',  ( 0.000000000000000000, 0.000000000000000000, -1.000000000000000000 ) ) ;
#2559=ADVANCED_FACE ( 'NONE', ( #2470 ), #12082, .F. ) ;
#2564=CARTESIAN_POINT ( 'NONE',  ( -9.354272893020521451, 2.499447352334152050, -47.88483805351501132 ) ) ;
#2568=EDGE_CURVE ( 'NONE', #12049, #13513, #12315, .T. ) ;
#2569=CARTESIAN_POINT ( 'NONE',  ( -24.73111225919155132, -6.857688092579577344, 47.70917337021941762 ) ) ;
#2571=EDGE_CURVE ( 'NONE', #6801, #1961, #12080, .T. ) ;
#2573=ORIENTED_EDGE ( 'NONE', *, *, #8609, .F. ) ;
#2582=CARTESIAN_POINT ( 'NONE',  ( -24.73660316015754290, -6.848489080522048411, 47.70033363922482295 ) ) ;
#2584=ORIENTED_EDGE ( 'NONE', *, *, #1928, .T. ) ;
#2585=DIRECTION ( 'NONE',  ( 0.8656763553492972108, 0.5006040828730397019, 1.548731138869852323E-14 ) ) ;
#2587=EDGE_CURVE ( 'NONE', #11281, #7187, #14290, .T. ) ;
#2592=ADVANCED_FACE ( 'NONE', ( #5299 ), #14280, .F. ) ;
#2593=LINE ( 'NONE', #1515, #4749 ) ;
#2595=CARTESIAN_POINT ( 'NONE',  ( -22.45192840590307881, 4.946501455397934954, 48.38495513066926890 ) ) ;
#2596=CARTESIAN_POINT ( 'NONE',  ( -7.999999999999986677, -2.249290599286305259, -58.00000000000012079 ) ) ;
#2612=CARTESIAN_POINT ( 'NONE',  ( -1.197457146693678753, -2.220571218158920335, -58.00000000000012079 ) ) ;
#2617=DIRECTION ( 'NONE',  ( 0.000000000000000000, 0.000000000000000000, -1.000000000000000000 ) ) ;
#2626=CIRCLE ( 'NONE', #413, 4.165819364273509962 ) ;
#2631=CARTESIAN_POINT ( 'NONE',  ( -9.084028622109864060, 2.040253803610913685, -48.06338840812200175 ) ) ;
#2633=CIRCLE ( 'NONE', #13439, 8.500000000000000000 ) ;
#2637=CARTESIAN_POINT ( 'NONE',  ( -24.60511756109301373, -7.062218017875619758, 48.00656353678737531 ) ) ;
#2638=EDGE_CURVE ( 'NONE', #11723, #4976, #458, .T. ) ;
#2648=CARTESIAN_POINT ( 'NONE',  ( -5.290523468902621929, 4.522075770548486418, 57.50000000000012079 ) ) ;
#2649=AXIS2_PLACEMENT_3D ( 'NONE', #5393, #14773, #8928 ) ;
#2660=ORIENTED_EDGE ( 'NONE', *, *, #1619, .T. ) ;
#2661=CARTESIAN_POINT ( 'NONE',  ( -5.040221427466104132, 4.089237592873841365, -48.50000000000012079 ) ) ;
#2664=VERTEX_POINT ( 'NONE', #3988 ) ;
#2665=CARTESIAN_POINT ( 'NONE',  ( -16.99999999999998579, -2.249290599286303927, -47.31370849898487307 ) ) ;
#2666=EDGE_LOOP ( 'NONE', ( #12457, #12075, #3735, #12990 ) ) ;
#2671=ORIENTED_EDGE ( 'NONE', *, *, #6671, .F. ) ;
#2673=CARTESIAN_POINT ( 'NONE',  ( -21.85476584171713199, 5.329050157244537900, 48.50000000000012079 ) ) ;
#2678=ORIENTED_EDGE ( 'NONE', *, *, #5771, .T. ) ;
#2687=DIRECTION ( 'NONE',  ( 1.000000000000000000, 0.000000000000000000, 0.000000000000000000 ) ) ;
#2692=AXIS2_PLACEMENT_3D ( 'NONE', #13877, #2254, #4722 ) ;
#2694=DIRECTION ( 'NONE',  ( -0.000000000000000000, -0.000000000000000000, 1.000000000000000000 ) ) ;
#2695=LINE ( 'NONE', #241, #11374 ) ;
#2696=ORIENTED_EDGE ( 'NONE', *, *, #3785, .T. ) ;
#2703=ORIENTED_EDGE ( 'NONE', *, *, #2920, .T. ) ;
#2707=ADVANCED_FACE ( 'NONE', ( #11342 ), #10099, .T. ) ;
#2708=CARTESIAN_POINT ( 'NONE',  ( -12.00298721683875236, -9.736506449376861383, -48.44214661497220931 ) ) ;
#2715=CARTESIAN_POINT ( 'NONE',  ( -8.787473000605775297, 2.499856724880853864, 48.43453164808066447 ) ) ;
#2721=ADVANCED_FACE ( 'NONE', ( #10284 ), #1980, .T. ) ;
#2725=EDGE_CURVE ( 'NONE', #4463, #10987, #10341, .T. ) ;
#2730=ORIENTED_EDGE ( 'NONE', *, *, #5696, .T. ) ;
#2735=TOROIDAL_SURFACE ( 'NONE', #11317, 8.500000000000000000, 0.5000000000000000000 ) ;
#2736=CARTESIAN_POINT ( 'NONE',  ( -11.54807159409575235, -9.445082653969818054, 48.38495513067856280 ) ) ;
#2748=VECTOR ( 'NONE', #8244, 1000.000000000000000 ) ;
#2752=VECTOR ( 'NONE', #13088, 1000.000000000000000 ) ;
#2765=ORIENTED_EDGE ( 'NONE', *, *, #1326, .T. ) ;
#2771=CARTESIAN_POINT ( 'NONE',  ( -25.15752072101212278, 2.619472661158555038, 48.00000000000012079 ) ) ;
#2772=CARTESIAN_POINT ( 'NONE',  ( -9.037775043065352065, 2.932694901963889489, -57.50000000000012079 ) ) ;
#2773=DIRECTION ( 'NONE',  ( 0.5006040828730242698, -0.8656763553493063146, 0.000000000000000000 ) ) ;
#2788=CIRCLE ( 'NONE', #14343, 9.000000000000001776 ) ;
#2790=AXIS2_PLACEMENT_3D ( 'NONE', #9319, #842, #14014 ) ;
#2793=EDGE_CURVE ( 'NONE', #10204, #6843, #7404, .T. ) ;
#2795=ADVANCED_FACE ( 'NONE', ( #11496 ), #13974, .T. ) ;
#2798=CARTESIAN_POINT ( 'NONE',  ( -16.99999999999998579, -2.249290599286303927, 50.50000000000012079 ) ) ;
#2800=CARTESIAN_POINT ( 'NONE',  ( -5.040221427466046400, 4.089237592873870675, -48.50000000000012079 ) ) ;
#2806=DIRECTION ( 'NONE',  ( 1.000000000000000000, -3.565820478396769525E-15, 0.000000000000000000 ) ) ;
#2808=ORIENTED_EDGE ( 'NONE', *, *, #13184, .T. ) ;
#2809=CYLINDRICAL_SURFACE ( 'NONE', #1473, 9.000000000000001776 ) ;
#2822=ORIENTED_EDGE ( 'NONE', *, *, #284, .T. ) ;
#2826=ORIENTED_EDGE ( 'NONE', *, *, #8884, .F. ) ;
#2833=ADVANCED_FACE ( 'NONE', ( #4811 ), #15216, .F. ) ;
#2834=CARTESIAN_POINT ( 'NONE',  ( -32.80254285330626374, -2.278009980413908231, -48.50000000000012079 ) ) ;
#2835=ORIENTED_EDGE ( 'NONE', *, *, #8, .T. ) ;
#2850=CARTESIAN_POINT ( 'NONE',  ( -10.14179456814604130, -8.352437357651758987, -48.12676452506694602 ) ) ;
#2861=AXIS2_PLACEMENT_3D ( 'NONE', #9230, #2375, #4530 ) ;
#2870=CARTESIAN_POINT ( 'NONE',  ( -24.91597137788995298, -6.538835002183793321, -48.06338840812244939 ) ) ;
#2874=CARTESIAN_POINT ( 'NONE',  ( -16.99999999999998579, -2.249290599286303927, -58.00000000000012079 ) ) ;
#2879=AXIS2_PLACEMENT_3D ( 'NONE', #6550, #9814, #10100 ) ;
#2880=ORIENTED_EDGE ( 'NONE', *, *, #9276, .T. ) ;
#2889=PRODUCT ( 'Plastic-Headed Retaining Pin', 'Plastic-Headed Retaining Pin', '', ( #4939 ) ) ;
#2894=ORIENTED_EDGE ( 'NONE', *, *, #4315, .T. ) ;
#2897=EDGE_LOOP ( 'NONE', ( #7244, #6551, #9686, #6560 ) ) ;
#2898=VERTEX_POINT ( 'NONE', #7270 ) ;
#2901=ORIENTED_EDGE ( 'NONE', *, *, #9974, .F. ) ;
#2910=ORIENTED_EDGE ( 'NONE', *, *, #6357, .F. ) ;
#2914=CARTESIAN_POINT ( 'NONE',  ( -3.190546569013415379, 0.8906624217387615339, -48.00000000000012079 ) ) ;
#2917=ORIENTED_EDGE ( 'NONE', *, *, #13409, .F. ) ;
#2919=CIRCLE ( 'NONE', #10797, 3.694885682588112896 ) ;
#2920=EDGE_CURVE ( 'NONE', #8990, #10817, #14526, .T. ) ;
#2929=AXIS2_PLACEMENT_3D ( 'NONE', #3710, #4720, #2484 ) ;
#2930=EDGE_CURVE ( 'NONE', #7613, #1961, #11081, .T. ) ;
#2935=CARTESIAN_POINT ( 'NONE',  ( -10.97058782713534164, -9.028420861780718454, -48.26891069786831423 ) ) ;
#2936=CARTESIAN_POINT ( 'NONE',  ( -9.268887740808379405, 2.359106894006888666, 47.70917337021941762 ) ) ;
#2940=AXIS2_PLACEMENT_3D ( 'NONE', #11432, #7760, #11285 ) ;
#2946=DIRECTION ( 'NONE',  ( -0.8420378618367723167, -0.5394184268574414576, -0.000000000000000000 ) ) ;
#2947=B_SPLINE_CURVE_WITH_KNOTS ( 'NONE', 3,
 ( #9612, #8376, #14294, #14378, #8461, #13144, #2595, #2673 ),
 .UNSPECIFIED., .F., .F.,
 ( 4, 2, 2, 4 ),
 ( 5.291795217412410304E-17, 0.001077686929059509672, 0.002155373858118966434, 0.004310747716237871285 ),
 .UNSPECIFIED. ) ;
#2956=CARTESIAN_POINT ( 'NONE',  ( -24.60804510916187837, -7.057608296800744085, -47.99579695943414492 ) ) ;
#2957=EDGE_CURVE ( 'NONE', #12265, #3301, #14572, .T. ) ;
#2961=CARTESIAN_POINT ( 'NONE',  ( -25.21252699837112132, -6.998437922861946880, 48.50000000000012079 ) ) ;
#2962=CARTESIAN_POINT ( 'NONE',  ( -16.99999999999998579, -2.249290599286303927, 48.00000000000012079 ) ) ;
#2971=AXIS2_PLACEMENT_3D ( 'NONE', #7820, #4420, #12506 ) ;
#2983=ADVANCED_FACE ( 'NONE', ( #7646 ), #6403, .F. ) ;
#2984=CIRCLE ( 'NONE', #6414, 0.5000000000000000000 ) ;
#2997=CARTESIAN_POINT ( 'NONE',  ( -1.197457146693678531, -2.220571218158920779, 48.50000000000012079 ) ) ;
#2998=ORIENTED_EDGE ( 'NONE', *, *, #7311, .T. ) ;
#3003=VERTEX_POINT ( 'NONE', #14637 ) ;
#3010=CARTESIAN_POINT ( 'NONE',  ( -12.14523415828296216, -9.827631355817223024, -48.50000000000012079 ) ) ;
#3023=CARTESIAN_POINT ( 'NONE',  ( -8.787473001628836045, 2.499856724289236887, 48.50000000000012079 ) ) ;
#3029=AXIS2_PLACEMENT_3D ( 'NONE', #7140, #7066, #11599 ) ;
#3030=EDGE_CURVE ( 'NONE', #9111, #6074, #9623, .T. ) ;
#3034=( BOUNDED_SURFACE ( )  B_SPLINE_SURFACE ( 3, 2, ( 
 ( #11855, #14172, #14326 ),
 ( #1390, #385, #6023 ),
 ( #164, #3774, #5081 ),
 ( #244, #9787, #3920 ),
 ( #8615, #13313, #13250 ),
 ( #9564, #3625, #3698 ),
 ( #9718, #14399, #8403 ),
 ( #8482, #3841, #7473 ) ),
 .UNSPECIFIED., .F., .F., .F. ) 
 B_SPLINE_SURFACE_WITH_KNOTS ( ( 4, 2, 2, 4 ),
 ( 3, 3 ),
 ( 0.000000000000000000, 0.001129222206655581574, 0.002258444413311163149, 0.004516888826622326297 ),
 ( 0.000000000000000000, 1.000000000000000000 ),
 .UNSPECIFIED. ) 
 GEOMETRIC_REPRESENTATION_ITEM ( )  RATIONAL_B_SPLINE_SURFACE ( (
 ( 1.000000000000000000, 0.7071067811864936159, 1.000000000000000000),
 ( 1.000000000000000000, 0.7608707698420138499, 1.000000000000000000),
 ( 1.000000000000000000, 0.8047257278452277784, 1.000000000000000000),
 ( 1.000000000000000000, 0.8783509392183566078, 1.000000000000000000),
 ( 1.000000000000000000, 0.9081758943102266057, 1.000000000000000000),
 ( 1.000000000000000000, 0.9781389570711758186, 1.000000000000000000),
 ( 1.000000000000000000, 0.9996704379314563793, 1.000000000000000000),
 ( 1.000000000000000000, 1.000000000000000000, 1.000000000000000000) ) ) 
 REPRESENTATION_ITEM ( '' )  SURFACE ( )  );
#3049=CARTESIAN_POINT ( 'NONE',  ( 0.5043391135745837195, 0.8906624217387615339, -48.50000000000012079 ) ) ;
#3061=CARTESIAN_POINT ( 'NONE',  ( -12.00298721683875236, -9.736506449376861383, 48.44214661497220931 ) ) ;
#3062=VERTEX_POINT ( 'NONE', #10422 ) ;
#3063=FACE_OUTER_BOUND ( 'NONE', #13077, .T. ) ;
#3065=CARTESIAN_POINT ( 'NONE',  ( -25.21252699837112132, -6.998437922861946880, -48.50000000000012079 ) ) ;
#3073=ORIENTED_EDGE ( 'NONE', *, *, #10860, .T. ) ;
#3090=TOROIDAL_SURFACE ( 'NONE', #6523, 3.694885682587998765, 0.5000000000000000000 ) ;
#3091=DIRECTION ( 'NONE',  ( -0.000000000000000000, 0.000000000000000000, 1.000000000000000000 ) ) ;
#3098=VECTOR ( 'NONE', #3632, 1000.000000000000000 ) ;
#3100=DIRECTION ( 'NONE',  ( 1.000000000000000000, 0.000000000000000000, 0.000000000000000000 ) ) ;
#3111=AXIS2_PLACEMENT_3D ( 'NONE', #10141, #9059, #14828 ) ;
#3112=CIRCLE ( 'NONE', #10985, 0.5000000000000000000 ) ;
#3119=DIRECTION ( 'NONE',  ( 0.000000000000000000, 0.000000000000000000, 1.000000000000000000 ) ) ;
#3120=CARTESIAN_POINT ( 'NONE',  ( -24.65452791727695114, 3.133494033999976391, -48.02161282446748203 ) ) ;
#3125=FACE_OUTER_BOUND ( 'NONE', #601, .T. ) ;
#3130=CARTESIAN_POINT ( 'NONE',  ( -8.842479278987921631, -7.118053859731281463, -47.50000000000012079 ) ) ;
#3137=ORIENTED_EDGE ( 'NONE', *, *, #12288, .F. ) ;
#3140=DIRECTION ( 'NONE',  ( 1.000000000000000000, 0.000000000000000000, 0.000000000000000000 ) ) ;
#3141=CARTESIAN_POINT ( 'NONE',  ( -10.99067925302910176, -8.982598353005794678, 48.14374739243442747 ) ) ;
#3143=AXIS2_PLACEMENT_3D ( 'NONE', #10152, #6834, #10305 ) ;
#3147=DIRECTION ( 'NONE',  ( 1.000000000000000000, 0.000000000000000000, 0.000000000000000000 ) ) ;
#3149=ORIENTED_EDGE ( 'NONE', *, *, #5378, .T. ) ;
#3152=CARTESIAN_POINT ( 'NONE',  ( -23.00932074697458773, 4.484017154434125629, -48.14374739243680068 ) ) ;
#3153=EDGE_CURVE ( 'NONE', #8990, #4595, #3176, .T. ) ;
#3162=ORIENTED_EDGE ( 'NONE', *, *, #2568, .T. ) ;
#3166=CARTESIAN_POINT ( 'NONE',  ( -30.80945343098651890, -5.389243620311580329, -58.00000000000012079 ) ) ;
#3174=FACE_OUTER_BOUND ( 'NONE', #12005, .T. ) ;
#3175=CARTESIAN_POINT ( 'NONE',  ( -16.99999999999998579, -2.249290599286303927, -48.00000000000012079 ) ) ;
#3176=CIRCLE ( 'NONE', #8816, 9.500000000000001776 ) ;
#3180=FACE_OUTER_BOUND ( 'NONE', #7828, .T. ) ;
#3183=CARTESIAN_POINT ( 'NONE',  ( -21.16581936427349575, -2.249290599286304371, -50.00000000000012079 ) ) ;
#3187=VECTOR ( 'NONE', #7429, 1000.000000000000000 ) ;
#3193=EDGE_CURVE ( 'NONE', #3752, #11723, #5389, .T. ) ;
#3201=EDGE_CURVE ( 'NONE', #2664, #7882, #12514, .T. ) ;
#3208=DIRECTION ( 'NONE',  ( -0.000000000000000000, -0.000000000000000000, 1.000000000000000000 ) ) ;
#3212=DIRECTION ( 'NONE',  ( 0.000000000000000000, 0.000000000000000000, -1.000000000000000000 ) ) ;
#3214=DIRECTION ( 'NONE',  ( 1.000000000000000000, 0.000000000000000000, 0.000000000000000000 ) ) ;
#3215=AXIS2_PLACEMENT_3D ( 'NONE', #6235, #10923, #372 ) ;
#3216=CARTESIAN_POINT ( 'NONE',  ( -10.31821280924931372, -8.288623256088383684, 47.74919337097148286 ) ) ;
#3222=CARTESIAN_POINT ( 'NONE',  ( -25.15752072101212278, 2.619472661158555038, 47.50000000000012079 ) ) ;
#3230=ORIENTED_EDGE ( 'NONE', *, *, #2793, .F. ) ;
#3233=DIRECTION ( 'NONE',  ( 0.000000000000000000, -0.000000000000000000, -1.000000000000000000 ) ) ;
#3237=AXIS2_PLACEMENT_3D ( 'NONE', #9408, #10327, #15021 ) ;
#3239=AXIS2_PLACEMENT_3D ( 'NONE', #13771, #7932, #15159 ) ;
#3242=DIRECTION ( 'NONE',  ( 1.000000000000000000, 0.000000000000000000, 0.000000000000000000 ) ) ;
#3246=VERTEX_POINT ( 'NONE', #7178 ) ;
#3254=CARTESIAN_POINT ( 'NONE',  ( -3.190546569013415379, 0.8906624217387615339, 48.00000000000012079 ) ) ;
#3258=DIRECTION ( 'NONE',  ( -1.000000000000000000, 0.000000000000000000, 0.000000000000000000 ) ) ;
#3276=VECTOR ( 'NONE', #10833, 1000.000000000000000 ) ;
#3285=DIRECTION ( 'NONE',  ( 0.000000000000000000, 0.000000000000000000, -1.000000000000000000 ) ) ;
#3287=DIRECTION ( 'NONE',  ( 0.5125013958363124900, 0.8586863916854809986, 0.000000000000000000 ) ) ;
#3288=DIRECTION ( 'NONE',  ( 1.000000000000000000, 0.000000000000000000, 0.000000000000000000 ) ) ;
#3289=CIRCLE ( 'NONE', #9903, 0.5000000000000004441 ) ;
#3292=EDGE_CURVE ( 'NONE', #14061, #1375, #14335, .T. ) ;
#3298=DIRECTION ( 'NONE',  ( 0.000000000000000000, 0.000000000000000000, -1.000000000000000000 ) ) ;
#3301=VERTEX_POINT ( 'NONE', #6394 ) ;
#3311=CARTESIAN_POINT ( 'NONE',  ( -0.9277479332649583021, -2.641590149077306826, 48.00000000000012079 ) ) ;
#3319=ORIENTED_EDGE ( 'NONE', *, *, #9565, .T. ) ;
#3350=CARTESIAN_POINT ( 'NONE',  ( -9.456839514482961562, 2.659958822950721835, -48.50000000000012079 ) ) ;
#3355=VERTEX_POINT ( 'NONE', #13258 ) ;
#3357=AXIS2_PLACEMENT_3D ( 'NONE', #11375, #10309, #5542 ) ;
#3359=LINE ( 'NONE', #1050, #495 ) ;
#3360=CIRCLE ( 'NONE', #11449, 9.000000000000001776 ) ;
#3375=CARTESIAN_POINT ( 'NONE',  ( -21.85476584171713199, 5.329050157244537900, -57.50000000000012079 ) ) ;
#3389=CARTESIAN_POINT ( 'NONE',  ( -16.99999999999998579, -2.249290599286303927, -38.00000000000012079 ) ) ;
#3400=CIRCLE ( 'NONE', #892, 5.165819364273509073 ) ;
#3403=DIRECTION ( 'NONE',  ( 1.000000000000000000, 0.000000000000000000, 0.000000000000000000 ) ) ;
#3407=FACE_OUTER_BOUND ( 'NONE', #11403, .T. ) ;
#3412=CARTESIAN_POINT ( 'NONE',  ( -25.01741698508091005, -6.338425579613558014, -47.50000000000012079 ) ) ;
#3413=CYLINDRICAL_SURFACE ( 'NONE', #6426, 9.000000000000001776 ) ;
#3414=EDGE_CURVE ( 'NONE', #2105, #13865, #6856, .T. ) ;
#3417=EDGE_CURVE ( 'NONE', #11292, #8222, #4227, .T. ) ;
#3418=ORIENTED_EDGE ( 'NONE', *, *, #9385, .T. ) ;
#3428=DIRECTION ( 'NONE',  ( 1.000000000000000000, 0.000000000000000000, 0.000000000000000000 ) ) ;
#3430=ADVANCED_FACE ( 'NONE', ( #15013, #13544 ), #12703, .F. ) ;
#3438=AXIS2_PLACEMENT_3D ( 'NONE', #3947, #15222, #10895 ) ;
#3447=CARTESIAN_POINT ( 'NONE',  ( -24.80190064845255193, -6.760980556683136911, -48.50000000000010658 ) ) ;
#3450=CARTESIAN_POINT ( 'NONE',  ( -11.55417588973486609, -9.448993130794820061, 48.32458034489290100 ) ) ;
#3452=EDGE_CURVE ( 'NONE', #170, #7882, #763, .T. ) ;
#3454=CYLINDRICAL_SURFACE ( 'NONE', #2166, 4.194885682587998765 ) ;
#3464=CARTESIAN_POINT ( 'NONE',  ( -25.21252699837112132, -6.998437922861946880, -58.00000000000012079 ) ) ;
#3468=DIRECTION ( 'NONE',  ( -0.8656763553492632379, -0.5006040828730989878, 1.736819309459606431E-15 ) ) ;
#3474=AXIS2_PLACEMENT_3D ( 'NONE', #4350, #12670, #12598 ) ;
#3475=ORIENTED_EDGE ( 'NONE', *, *, #9530, .F. ) ;
#3488=EDGE_CURVE ( 'NONE', #3759, #3805, #14242, .T. ) ;
#3489=CARTESIAN_POINT ( 'NONE',  ( -11.83418063572647760, -2.249290599286303927, -57.50000000000012079 ) ) ;
#3491=CARTESIAN_POINT ( 'NONE',  ( -24.95893038578871881, -6.453098109823664608, -47.50000000000011369 ) ) ;
#3496=CARTESIAN_POINT ( 'NONE',  ( -3.190546569013415379, 0.8906624217387615339, 58.00000000000012079 ) ) ;
#3497=ORIENTED_EDGE ( 'NONE', *, *, #11424, .F. ) ;
#3503=CYLINDRICAL_SURFACE ( 'NONE', #4597, 0.5000000000000004441 ) ;
#3509=FACE_OUTER_BOUND ( 'NONE', #2666, .T. ) ;
#3511=CARTESIAN_POINT ( 'NONE',  ( -25.27051402993791029, -6.915952606384455414, 48.19241902544784750 ) ) ;
#3518=CIRCLE ( 'NONE', #6700, 9.000000000000001776 ) ;
#3527=EDGE_LOOP ( 'NONE', ( #8071, #1453, #1730, #11947 ) ) ;
#3530=CARTESIAN_POINT ( 'NONE',  ( -24.54316048551696028, -7.158540021523408292, -48.50000000000011369 ) ) ;
#3537=ORIENTED_EDGE ( 'NONE', *, *, #6762, .T. ) ;
#3556=CARTESIAN_POINT ( 'NONE',  ( -11.55417588973486609, -9.448993130794820061, -48.32458034489290100 ) ) ;
#3560=CARTESIAN_POINT ( 'NONE',  ( -25.46282903980762669, -6.565599745187292946, 48.00000000000012079 ) ) ;
#3562=DIRECTION ( 'NONE',  ( 1.000000000000000000, 0.000000000000000000, 0.000000000000000000 ) ) ;
#3566=VERTEX_POINT ( 'NONE', #6397 ) ;
#3578=CARTESIAN_POINT ( 'NONE',  ( -25.15752072101212278, 2.619472661158555038, -47.50000000000012079 ) ) ;
#3586=ORIENTED_EDGE ( 'NONE', *, *, #4794, .F. ) ;
#3606=ORIENTED_EDGE ( 'NONE', *, *, #9614, .F. ) ;
#3607=CARTESIAN_POINT ( 'NONE',  ( -8.593267841128518825, 2.185894787177926624, 48.01308457333531265 ) ) ;
#3609=ORIENTED_EDGE ( 'NONE', *, *, #11279, .T. ) ;
#3610=CARTESIAN_POINT ( 'NONE',  ( -22.54958699671023581, 4.838095916862976686, -48.21133583021728697 ) ) ;
#3612=ORIENTED_EDGE ( 'NONE', *, *, #7311, .F. ) ;
#3625=CARTESIAN_POINT ( 'NONE',  ( -23.00932074697458773, 4.484017154434125629, 48.14374739243680068 ) ) ;
#3632=DIRECTION ( 'NONE',  ( 0.000000000000000000, 0.000000000000000000, -1.000000000000000000 ) ) ;
#3637=DIRECTION ( 'NONE',  ( -0.5006040828730974335, 0.8656763553492640151, 0.000000000000000000 ) ) ;
#3649=ADVANCED_FACE ( 'NONE', ( #12944 ), #9401, .T. ) ;
#3651=ADVANCED_FACE ( 'NONE', ( #6827 ), #12031, .T. ) ;
#3658=CARTESIAN_POINT ( 'NONE',  ( -16.99999999999998579, -2.249290599286303927, -48.00000000000012079 ) ) ;
#3662=CARTESIAN_POINT ( 'NONE',  ( -24.89252171451660445, -6.585377854361484040, 48.09696226170979827 ) ) ;
#3667=DIRECTION ( 'NONE',  ( 0.000000000000000000, 0.000000000000000000, -1.000000000000000000 ) ) ;
#3670=EDGE_CURVE ( 'NONE', #7624, #3759, #11359, .T. ) ;
#3672=LINE ( 'NONE', #4518, #8667 ) ;
#3674=DIRECTION ( 'NONE',  ( -0.8908241094534361526, -0.4543483311474716957, 0.000000000000000000 ) ) ;
#3680=DIRECTION ( 'NONE',  ( 1.000000000000000000, -8.673617379884027583E-15, 0.000000000000000000 ) ) ;
#3682=FACE_OUTER_BOUND ( 'NONE', #4540, .T. ) ;
#3687=CARTESIAN_POINT ( 'NONE',  ( 0.5043391135745837195, 0.8906624217387615339, 48.50000000000012079 ) ) ;
#3688=VERTEX_POINT ( 'NONE', #3065 ) ;
#3698=CARTESIAN_POINT ( 'NONE',  ( -23.03920594196030791, 4.522656845271360915, 48.26696389624889605 ) ) ;
#3701=CARTESIAN_POINT ( 'NONE',  ( -25.01741698508091005, -6.338425579613558014, 47.50000000000012079 ) ) ;
#3706=DIRECTION ( 'NONE',  ( 1.000000000000000000, 0.000000000000000000, 0.000000000000000000 ) ) ;
#3707=AXIS2_PLACEMENT_3D ( 'NONE', #956, #5668, #4503 ) ;
#3710=CARTESIAN_POINT ( 'NONE',  ( -28.95977857253358323, -8.587818791446789390, -57.50000000000012079 ) ) ;
#3715=AXIS2_PLACEMENT_3D ( 'NONE', #14322, #12157, #8829 ) ;
#3716=CARTESIAN_POINT ( 'NONE',  ( -16.99999999999998579, -2.249290599286303927, 47.50000000000012079 ) ) ;
#3725=DIRECTION ( 'NONE',  ( 0.8656763553492639041, 0.5006040828730973224, 0.000000000000000000 ) ) ;
#3726=CIRCLE ( 'NONE', #4205, 4.000000000000000000 ) ;
#3727=EDGE_CURVE ( 'NONE', #8849, #7744, #3924, .T. ) ;
#3735=ORIENTED_EDGE ( 'NONE', *, *, #9530, .T. ) ;
#3736=DIRECTION ( 'NONE',  ( 0.000000000000000000, 0.000000000000000000, 1.000000000000000000 ) ) ;
#3743=ADVANCED_FACE ( 'NONE', ( #971 ), #12609, .F. ) ;
#3750=CIRCLE ( 'NONE', #14808, 4.165819364273509962 ) ;
#3752=VERTEX_POINT ( 'NONE', #4207 ) ;
#3759=VERTEX_POINT ( 'NONE', #8911 ) ;
#3762=CARTESIAN_POINT ( 'NONE',  ( -9.457494889590920550, -7.172893779636416056, 47.50000000000009237 ) ) ;
#3769=DIRECTION ( 'NONE',  ( -0.5006040828730773384, 0.8656763553492754504, 0.000000000000000000 ) ) ;
#3772=EDGE_LOOP ( 'NONE', ( #7830, #6299, #2660, #10697, #1963, #9747 ) ) ;
#3773=VECTOR ( 'NONE', #13976, 1000.000000000000114 ) ;
#3774=CARTESIAN_POINT ( 'NONE',  ( -24.38033816570045076, 2.914516366099690448, 47.90685900410169040 ) ) ;
#3781=ORIENTED_EDGE ( 'NONE', *, *, #485, .F. ) ;
#3782=SHAPE_DEFINITION_REPRESENTATION ( #6708, #8914 ) ;
#3785=EDGE_CURVE ( 'NONE', #13205, #2898, #14729, .T. ) ;
#3786=CARTESIAN_POINT ( 'NONE',  ( -9.198099345814858552, 2.262399347264687943, -48.43121057161710041 ) ) ;
#3787=CARTESIAN_POINT ( 'NONE',  ( -24.96222495693456978, -7.431276100536581275, 58.00000000000012079 ) ) ;
#3790=ADVANCED_FACE ( 'NONE', ( #8576 ), #14007, .F. ) ;
#3797=DIRECTION ( 'NONE',  ( 1.000000000000000000, 8.270659117969274159E-16, 0.000000000000000000 ) ) ;
#3798=DIRECTION ( 'NONE',  ( 1.000000000000000000, 0.000000000000000000, 0.000000000000000000 ) ) ;
#3805=VERTEX_POINT ( 'NONE', #2369 ) ;
#3817=ORIENTED_EDGE ( 'NONE', *, *, #10104, .F. ) ;
#3823=CARTESIAN_POINT ( 'NONE',  ( -28.70947653109703523, -9.020656969121422009, 57.50000000000012079 ) ) ;
#3825=CARTESIAN_POINT ( 'NONE',  ( -22.41471376588497222, 4.941665658445489662, 48.26816462195809265 ) ) ;
#3826=EDGE_LOOP ( 'NONE', ( #14610, #2703, #71 ) ) ;
#3831=EDGE_LOOP ( 'NONE', ( #10010, #12858, #6498, #1677 ) ) ;
#3838=LINE ( 'NONE', #13018, #4196 ) ;
#3839=DIRECTION ( 'NONE',  ( -0.000000000000000000, -0.000000000000000000, 1.000000000000000000 ) ) ;
#3841=CARTESIAN_POINT ( 'NONE',  ( -21.85476584171706449, 5.329050157244580532, 48.50000000000012079 ) ) ;
#3844=CARTESIAN_POINT ( 'NONE',  ( -28.70947653109703168, -9.020656969121420232, 57.50000000000012079 ) ) ;
#3851=CARTESIAN_POINT ( 'NONE',  ( -8.729485970062036415, 2.417371407811747197, -48.19241902544784750 ) ) ;
#3862=ADVANCED_FACE ( 'NONE', ( #6275 ), #12066, .F. ) ;
#3865=ORIENTED_EDGE ( 'NONE', *, *, #6225, .T. ) ;
#3869=PRODUCT_DEFINITION_FORMATION_WITH_SPECIFIED_SOURCE ( 'ANY', '', #2889, .NOT_KNOWN. ) ;
#3870=DIRECTION ( 'NONE',  ( 0.8420378618367728718, 0.5394184268574404584, -0.000000000000000000 ) ) ;
#3872=VECTOR ( 'NONE', #4501, 1000.000000000000000 ) ;
#3879=CARTESIAN_POINT ( 'NONE',  ( -16.99999999999998579, -2.249290599286303927, -50.50000000000012079 ) ) ;
#3888=ORIENTED_EDGE ( 'NONE', *, *, #13193, .T. ) ;
#3889=CARTESIAN_POINT ( 'NONE',  ( -12.14523415828296216, -9.827631355817223024, 48.50000000000012079 ) ) ;
#3892=DIRECTION ( 'NONE',  ( 1.000000000000000000, 0.000000000000000000, 0.000000000000000000 ) ) ;
#3894=EDGE_LOOP ( 'NONE', ( #1837, #2359, #11373, #7836 ) ) ;
#3908=DIRECTION ( 'NONE',  ( 1.000000000000000000, 0.000000000000000000, 0.000000000000000000 ) ) ;
#3913=CIRCLE ( 'NONE', #13490, 8.500000000000000000 ) ;
#3917=EDGE_CURVE ( 'NONE', #6801, #6058, #8794, .T. ) ;
#3918=DIRECTION ( 'NONE',  ( 1.000000000000000000, 0.000000000000000000, 0.000000000000000000 ) ) ;
#3920=CARTESIAN_POINT ( 'NONE',  ( -24.14404371603619381, 3.605862562765568491, 48.08251050686933326 ) ) ;
#3924=CIRCLE ( 'NONE', #718, 4.194885682587998765 ) ;
#3935=CARTESIAN_POINT ( 'NONE',  ( -24.96222495693456978, -7.431276100536581275, 57.50000000000012079 ) ) ;
#3947=CARTESIAN_POINT ( 'NONE',  ( -16.99999999999998579, -2.249290599286303927, 38.00000000000012079 ) ) ;
#3951=ORIENTED_EDGE ( 'NONE', *, *, #8899, .F. ) ;
#3955=ADVANCED_FACE ( 'NONE', ( #14955 ), #3413, .T. ) ;
#3960=DIRECTION ( 'NONE',  ( 0.5394184268574402363, -0.8420378618367729828, 0.000000000000000000 ) ) ;
#3962=CYLINDRICAL_SURFACE ( 'NONE', #1794, 4.665819364273509073 ) ;
#3966=AXIS2_PLACEMENT_3D ( 'NONE', #8979, #1897, #14901 ) ;
#3970=EDGE_LOOP ( 'NONE', ( #14521, #4201, #1735, #2671 ) ) ;
#3974=ORIENTED_EDGE ( 'NONE', *, *, #7880, .F. ) ;
#3980=ORIENTED_EDGE ( 'NONE', *, *, #7921, .F. ) ;
#3982=ADVANCED_FACE ( 'NONE', ( #13795 ), #4709, .F. ) ;
#3984=CARTESIAN_POINT ( 'NONE',  ( -12.99999999999998757, -2.249290599286303927, -47.31370849898487307 ) ) ;
#3985=ORIENTED_EDGE ( 'NONE', *, *, #3452, .T. ) ;
#3986=VECTOR ( 'NONE', #15219, 1000.000000000000000 ) ;
#3988=CARTESIAN_POINT ( 'NONE',  ( -11.83418063572647760, -2.249290599286303927, -58.00000000000012079 ) ) ;
#3994=ORIENTED_EDGE ( 'NONE', *, *, #9732, .F. ) ;
#3995=CIRCLE ( 'NONE', #9672, 0.5000000000000004441 ) ;
#4006=AXIS2_PLACEMENT_3D ( 'NONE', #93, #2617, #4783 ) ;
#4007=CARTESIAN_POINT ( 'NONE',  ( -8.982583014919022446, 1.839844381040865118, 47.50000000000012079 ) ) ;
#4010=DIRECTION ( 'NONE',  ( -0.000000000000000000, 0.000000000000000000, 1.000000000000000000 ) ) ;
#4020=CARTESIAN_POINT ( 'NONE',  ( -25.46282903980763024, -6.565599745187293834, -48.00000000000012079 ) ) ;
#4025=CARTESIAN_POINT ( 'NONE',  ( -1.197457146693683194, -2.220571218158922999, -57.50000000000012079 ) ) ;
#4029=CYLINDRICAL_SURFACE ( 'NONE', #4832, 0.5000000000000002220 ) ;
#4042=CARTESIAN_POINT ( 'NONE',  ( -24.54250511040913096, 2.674312581063694516, 47.50000000000008527 ) ) ;
#4049=VERTEX_POINT ( 'NONE', #1731 ) ;
#4052=EDGE_CURVE ( 'NONE', #8396, #12161, #13505, .T. ) ;
#4056=CYLINDRICAL_SURFACE ( 'NONE', #9926, 0.5000000000000001110 ) ;
#4058=CIRCLE ( 'NONE', #2364, 4.194885682587998765 ) ;
#4067=CIRCLE ( 'NONE', #10976, 9.500000000000001776 ) ;
#4078=CARTESIAN_POINT ( 'NONE',  ( -9.148597373295839219, 2.167486929505451076, 48.18452149279841024 ) ) ;
#4082=CARTESIAN_POINT ( 'NONE',  ( 0.000000000000000000, 0.000000000000000000, 0.000000000000000000 ) ) ;
#4088=CARTESIAN_POINT ( 'NONE',  ( -16.99999999999998579, -2.249290599286303927, -38.00000000000012079 ) ) ;
#4089=CARTESIAN_POINT ( 'NONE',  ( -5.290523468902621929, 4.522075770548486418, -48.00000000000012079 ) ) ;
#4101=CARTESIAN_POINT ( 'NONE',  ( -25.21252699837112132, -6.998437922861944216, 48.36782213136056896 ) ) ;
#4103=TOROIDAL_SURFACE ( 'NONE', #10019, 1.000000000000000000, 0.5000000000000000000 ) ;
#4106=FACE_OUTER_BOUND ( 'NONE', #5346, .T. ) ;
#4107=ORIENTED_EDGE ( 'NONE', *, *, #3785, .F. ) ;
#4111=CIRCLE ( 'NONE', #6109, 3.694885682588112896 ) ;
#4115=CARTESIAN_POINT ( 'NONE',  ( -8.787473001628837821, 2.499856724289235554, -57.50000000000012079 ) ) ;
#4116=ORIENTED_EDGE ( 'NONE', *, *, #6408, .F. ) ;
#4127=DIRECTION ( 'NONE',  ( 0.5006040828730228265, -0.8656763553493070917, 0.000000000000000000 ) ) ;
#4128=CARTESIAN_POINT ( 'NONE',  ( -21.85476584171713199, 5.329050157244540564, -57.50000000000012079 ) ) ;
#4130=LINE ( 'NONE', #3984, #7179 ) ;
#4133=EDGE_CURVE ( 'NONE', #6293, #10292, #11323, .T. ) ;
#4136=CARTESIAN_POINT ( 'NONE',  ( -9.271822474830681671, -6.861803161813159413, 48.00000000000019895 ) ) ;
#4138=CARTESIAN_POINT ( 'NONE',  ( -21.66581936427349575, -2.249290599286304371, -50.50000000000012079 ) ) ;
#4140=ORIENTED_EDGE ( 'NONE', *, *, #1789, .T. ) ;
#4145=CARTESIAN_POINT ( 'NONE',  ( -16.99999999999998579, -2.249290599286303927, 57.50000000000012079 ) ) ;
#4146=CARTESIAN_POINT ( 'NONE',  ( -25.46282903980766932, -6.565599745187317815, -58.00000000000012079 ) ) ;
#4148=CIRCLE ( 'NONE', #2692, 0.4999999999999995559 ) ;
#4149=CARTESIAN_POINT ( 'NONE',  ( -3.285520523750506516, 5.681530634152946568, 48.50000000000012079 ) ) ;
#4151=CARTESIAN_POINT ( 'NONE',  ( -8.590985667557523797, 2.187759657648595368, -48.00000000000012079 ) ) ;
#4163=CARTESIAN_POINT ( 'NONE',  ( -24.54316048551696383, -7.158540021523408292, -48.37147253714708484 ) ) ;
#4165=CARTESIAN_POINT ( 'NONE',  ( -28.95977857253364007, -8.587818791446682809, -58.00000000000012079 ) ) ;
#4167=TOROIDAL_SURFACE ( 'NONE', #12296, 8.500000000000000000, 0.5000000000000000000 ) ;
#4173=LINE ( 'NONE', #8874, #3187 ) ;
#4176=DIRECTION ( 'NONE',  ( -0.000000000000000000, 0.000000000000000000, 1.000000000000000000 ) ) ;
#4177=AXIS2_PLACEMENT_3D ( 'NONE', #4589, #14638, #6716 ) ;
#4178=ORIENTED_EDGE ( 'NONE', *, *, #2571, .F. ) ;
#4179=CARTESIAN_POINT ( 'NONE',  ( -8.958610760419841057, 1.823307968896474840, 58.00000000000012079 ) ) ;
#4186=CARTESIAN_POINT ( 'NONE',  ( -12.14523415828296216, -9.827631355817223024, -48.50000000000012079 ) ) ;
#4194=ORIENTED_EDGE ( 'NONE', *, *, #12608, .T. ) ;
#4196=VECTOR ( 'NONE', #2694, 1000.000000000000000 ) ;
#4200=LINE ( 'NONE', #4128, #10170 ) ;
#4201=ORIENTED_EDGE ( 'NONE', *, *, #1326, .F. ) ;
#4205=AXIS2_PLACEMENT_3D ( 'NONE', #13603, #2057, #7756 ) ;
#4207=CARTESIAN_POINT ( 'NONE',  ( -28.70947653109703168, -9.020656969121420232, -57.50000000000012079 ) ) ;
#4213=ORIENTED_EDGE ( 'NONE', *, *, #6762, .F. ) ;
#4227=LINE ( 'NONE', #6617, #13746 ) ;
#4239=FACE_OUTER_BOUND ( 'NONE', #7810, .T. ) ;
#4246=AXIS2_PLACEMENT_3D ( 'NONE', #2997, #7535, #459 ) ;
#4248=CARTESIAN_POINT ( 'NONE',  ( -25.15752072101212278, 2.619472661158555038, -48.00000000000012079 ) ) ;
#4249=CARTESIAN_POINT ( 'NONE',  ( -25.34903703195771385, -6.790201970332132575, -48.06291368403887532 ) ) ;
#4251=AXIS2_PLACEMENT_3D ( 'NONE', #15205, #11579, #15130 ) ;
#4270=ORIENTED_EDGE ( 'NONE', *, *, #4521, .T. ) ;
#4273=DIRECTION ( 'NONE',  ( -0.5394184268574488961, 0.8420378618367674317, 0.000000000000000000 ) ) ;
#4275=CARTESIAN_POINT ( 'NONE',  ( -8.537170960192327129, 2.067018546614582508, -57.50000000000012079 ) ) ;
#4277=ORIENTED_EDGE ( 'NONE', *, *, #12708, .F. ) ;
#4278=PLANE ( 'NONE',  #4454 ) ;
#4280=DIRECTION ( 'NONE',  ( 0.000000000000000000, 0.000000000000000000, 1.000000000000000000 ) ) ;
#4286=EDGE_CURVE ( 'NONE', #4371, #3688, #5113, .T. ) ;
#4293=DIRECTION ( 'NONE',  ( 0.000000000000000000, 0.000000000000000000, 1.000000000000000000 ) ) ;
#4294=DIRECTION ( 'NONE',  ( -0.000000000000000000, -0.000000000000000000, 1.000000000000000000 ) ) ;
#4297=CARTESIAN_POINT ( 'NONE',  ( -28.70947653109703168, -9.020656969121420232, -48.50000000000012079 ) ) ;
#4307=ADVANCED_FACE ( 'NONE', ( #6344 ), #2500, .F. ) ;
#4309=( NAMED_UNIT ( * ) PLANE_ANGLE_UNIT ( ) SI_UNIT ( $, .RADIAN. ) );
#4312=CARTESIAN_POINT ( 'NONE',  ( -5.040221427466109461, 4.089237592873834259, -48.00000000000012079 ) ) ;
#4315=EDGE_CURVE ( 'NONE', #1125, #12049, #8436, .T. ) ;
#4316=DIRECTION ( 'NONE',  ( 0.000000000000000000, 0.000000000000000000, -1.000000000000000000 ) ) ;
#4322=CARTESIAN_POINT ( 'NONE',  ( -25.01741698508091005, -6.338425579613558014, -48.00000000000010658 ) ) ;
#4330=EDGE_LOOP ( 'NONE', ( #12931, #13996, #3781, #10676 ) ) ;
#4341=DIRECTION ( 'NONE',  ( -0.000000000000000000, 0.000000000000000000, 1.000000000000000000 ) ) ;
#4350=CARTESIAN_POINT ( 'NONE',  ( -3.190546569013415379, 0.8906624217387615339, 57.50000000000012079 ) ) ;
#4361=CARTESIAN_POINT ( 'NONE',  ( -3.190546569013415379, 0.8906624217387615339, -48.50000000000012079 ) ) ;
#4371=VERTEX_POINT ( 'NONE', #4297 ) ;
#4372=DIRECTION ( 'NONE',  ( -0.000000000000000000, -0.000000000000000000, 1.000000000000000000 ) ) ;
#4384=DIRECTION ( 'NONE',  ( 1.000000000000000000, 0.000000000000000000, 0.000000000000000000 ) ) ;
#4389=DIRECTION ( 'NONE',  ( 1.000000000000000000, 0.000000000000000000, 0.000000000000000000 ) ) ;
#4404=VECTOR ( 'NONE', #5477, 1000.000000000000000 ) ;
#4406=CARTESIAN_POINT ( 'NONE',  ( -16.99999999999998579, -2.249290599286303927, 58.00000000000012079 ) ) ;
#4412=ORIENTED_EDGE ( 'NONE', *, *, #13506, .T. ) ;
#4419=CARTESIAN_POINT ( 'NONE',  ( -16.99999999999998579, -2.249290599286303927, -38.50000000000012790 ) ) ;
#4420=DIRECTION ( 'NONE',  ( -0.000000000000000000, 0.000000000000000000, 1.000000000000000000 ) ) ;
#4423=EDGE_CURVE ( 'NONE', #7757, #14061, #2074, .T. ) ;
#4426=ADVANCED_FACE ( 'NONE', ( #11529 ), #986, .F. ) ;
#4427=DIRECTION ( 'NONE',  ( 0.000000000000000000, -1.000000000000000000, 0.000000000000000000 ) ) ;
#4431=DIRECTION ( 'NONE',  ( 0.000000000000000000, 0.000000000000000000, 1.000000000000000000 ) ) ;
#4432=DIRECTION ( 'NONE',  ( 0.000000000000000000, 0.000000000000000000, -1.000000000000000000 ) ) ;
#4442=DIRECTION ( 'NONE',  ( 0.000000000000000000, 0.000000000000000000, 1.000000000000000000 ) ) ;
#4444=AXIS2_PLACEMENT_3D ( 'NONE', #8867, #10964, #2806 ) ;
#4447=CARTESIAN_POINT ( 'NONE',  ( -9.875903985900574611, 2.387222743937553293, 58.00000000000012079 ) ) ;
#4454=AXIS2_PLACEMENT_3D ( 'NONE', #9061, #5373, #11209 ) ;
#4463=VERTEX_POINT ( 'NONE', #1714 ) ;
#4465=CARTESIAN_POINT ( 'NONE',  ( 1.004339113574583608, 0.8906624217387615339, 57.50000000000012079 ) ) ;
#4468=CARTESIAN_POINT ( 'NONE',  ( -9.035163663297472780, 1.943345362497546747, 48.01692658285808335 ) ) ;
#4469=EDGE_CURVE ( 'NONE', #2463, #3805, #13807, .T. ) ;
#4478=DIRECTION ( 'NONE',  ( 0.8586863916854811096, -0.5125013958363124900, 0.000000000000000000 ) ) ;
#4481=VECTOR ( 'NONE', #2514, 1000.000000000000000 ) ;
#4483=DIRECTION ( 'NONE',  ( 0.000000000000000000, 0.000000000000000000, 1.000000000000000000 ) ) ;
#4486=DIRECTION ( 'NONE',  ( -0.5394184268574404584, 0.8420378618367728718, 0.000000000000000000 ) ) ;
#4492=EDGE_LOOP ( 'NONE', ( #14314, #14476, #3985, #51 ) ) ;
#4498=FACE_OUTER_BOUND ( 'NONE', #3894, .T. ) ;
#4499=VECTOR ( 'NONE', #473, 1000.000000000000000 ) ;
#4501=DIRECTION ( 'NONE',  ( 0.8656763553493062036, 0.5006040828730242698, 0.000000000000000000 ) ) ;
#4503=DIRECTION ( 'NONE',  ( -0.5394184268574404584, 0.8420378618367728718, 0.000000000000000000 ) ) ;
#4518=CARTESIAN_POINT ( 'NONE',  ( -8.787473001628837821, 2.499856724289235554, 58.00000000000012079 ) ) ;
#4521=EDGE_CURVE ( 'NONE', #8826, #8112, #155, .T. ) ;
#4522=ORIENTED_EDGE ( 'NONE', *, *, #1661, .F. ) ;
#4530=DIRECTION ( 'NONE',  ( 1.000000000000000000, 0.000000000000000000, 0.000000000000000000 ) ) ;
#4531=ORIENTED_EDGE ( 'NONE', *, *, #8059, .T. ) ;
#4534=ORIENTED_EDGE ( 'NONE', *, *, #9772, .F. ) ;
#4538=LINE ( 'NONE', #2229, #532 ) ;
#4540=EDGE_LOOP ( 'NONE', ( #3612, #11674, #5172, #4213 ) ) ;
#4550=ORIENTED_EDGE ( 'NONE', *, *, #8059, .F. ) ;
#4555=EDGE_LOOP ( 'NONE', ( #12414, #6348, #1816 ) ) ;
#4559=EDGE_CURVE ( 'NONE', #9532, #11054, #11437, .T. ) ;
#4560=FACE_OUTER_BOUND ( 'NONE', #9113, .T. ) ;
#4565=CLOSED_SHELL ( 'NONE', ( #14401, #2983, #11773, #12992, #2175, #8693, #5751, #7583, #8199, #8258, #7530, #14137, #10883, #11752, #3982, #9541, #1097, #6779, #3955, #6097, #10036, #12337, #8648, #1643, #9208, #1868, #13139, #8984, #12408, #15005, #2125, #1662, #6516, #7354, #6133, #8438, #15049, #10067, #2833, #6549, #8456, #851, #5358, #5372, #2592, #7165, #8476, #8835, #8548, #2721, #1797, #10299, #2795, #10668, #2707, #6497, #10626, #13589, #10510, #14716, #6637, #12508, #3430, #12820, #13223, #3743, #14418, #8287, #202, #4809, #12520, #4426, #3649, #12462, #5082, #13809, #3790, #9474, #11976, #3862, #10790, #12253, #4307, #10167, #6316, #10370, #15201, #13369, #1621, #11925, #13628, #8590, #2559, #9235, #12482, #3651, #8660, #13463, #13461, #1952 ) ) ;
#4566=ORIENTED_EDGE ( 'NONE', *, *, #1579, .F. ) ;
#4571=DIRECTION ( 'NONE',  ( 0.000000000000000000, 0.000000000000000000, -1.000000000000000000 ) ) ;
#4579=FACE_OUTER_BOUND ( 'NONE', #1220, .T. ) ;
#4581=LINE ( 'NONE', #9281, #3773 ) ;
#4583=EDGE_LOOP ( 'NONE', ( #4116, #1006, #13937, #13292 ) ) ;
#4587=CIRCLE ( 'NONE', #6305, 4.194885682588113340 ) ;
#4589=CARTESIAN_POINT ( 'NONE',  ( -3.190546569013415379, 0.8906624217387615339, 48.50000000000012079 ) ) ;
#4595=VERTEX_POINT ( 'NONE', #9313 ) ;
#4597=AXIS2_PLACEMENT_3D ( 'NONE', #8206, #9668, #5897 ) ;
#4606=ORIENTED_EDGE ( 'NONE', *, *, #3292, .T. ) ;
#4611=VERTEX_POINT ( 'NONE', #6166 ) ;
#4616=EDGE_CURVE ( 'NONE', #10292, #9229, #5717, .T. ) ;
#4636=LINE ( 'NONE', #5955, #15057 ) ;
#4641=DIRECTION ( 'NONE',  ( -0.000000000000000000, 1.000000000000000000, 0.000000000000000000 ) ) ;
#4649=B_SPLINE_CURVE_WITH_KNOTS ( 'NONE', 3,
 ( #14770, #6326, #469, #5312, #396, #14618, #12098, #1625, #8847, #14551, #2708, #3010 ),
 .UNSPECIFIED., .F., .F.,
 ( 4, 2, 2, 2, 2, 4 ),
 ( 0.000000000000000000, 0.001071381053236907443, 0.002142762106473816621, 0.003214143159710726016, 0.003749833686329184183, 0.004285524212947642783 ),
 .UNSPECIFIED. ) ;
#4657=CIRCLE ( 'NONE', #10058, 0.5000000000000001110 ) ;
#4659=DIRECTION ( 'NONE',  ( 0.000000000000000000, -0.000000000000000000, -1.000000000000000000 ) ) ;
#4663=EDGE_LOOP ( 'NONE', ( #14324, #9179, #677 ) ) ;
#4673=EDGE_CURVE ( 'NONE', #1961, #7398, #13817, .T. ) ;
#4674=CARTESIAN_POINT ( 'NONE',  ( -16.99999999999998579, -2.249290599286303927, -58.00000000000012079 ) ) ;
#4682=ORIENTED_EDGE ( 'NONE', *, *, #10425, .F. ) ;
#4692=FACE_OUTER_BOUND ( 'NONE', #5342, .T. ) ;
#4701=DIRECTION ( 'NONE',  ( -0.000000000000000000, 0.000000000000000000, 1.000000000000000000 ) ) ;
#4702=CARTESIAN_POINT ( 'NONE',  ( -16.99999999999998579, -2.249290599286303927, -50.00000000000012079 ) ) ;
#4705=AXIS2_PLACEMENT_3D ( 'NONE', #14154, #11835, #6996 ) ;
#4706=ORIENTED_EDGE ( 'NONE', *, *, #4933, .F. ) ;
#4707=FACE_OUTER_BOUND ( 'NONE', #10747, .T. ) ;
#4708=FACE_OUTER_BOUND ( 'NONE', #1940, .T. ) ;
#4709=TOROIDAL_SURFACE ( 'NONE', #6911, 9.500000000000001776, 0.5000000000000000000 ) ;
#4711=CARTESIAN_POINT ( 'NONE',  ( -11.57001547143821085, -9.459140135624386048, -48.26605223432068925 ) ) ;
#4717=EDGE_CURVE ( 'NONE', #170, #7490, #310, .T. ) ;
#4718=EDGE_CURVE ( 'NONE', #14789, #60, #10881, .T. ) ;
#4719=VECTOR ( 'NONE', #1723, 1000.000000000000000 ) ;
#4720=DIRECTION ( 'NONE',  ( 0.8656763553492632379, 0.5006040828730989878, 1.736819309459606431E-15 ) ) ;
#4722=DIRECTION ( 'NONE',  ( -0.5394184268574385710, 0.8420378618367740930, 0.000000000000000000 ) ) ;
#4728=CARTESIAN_POINT ( 'NONE',  ( -21.58505662828840244, 4.908031226326156293, 58.00000000000012079 ) ) ;
#4730=CARTESIAN_POINT ( 'NONE',  ( -22.16581936427349575, -2.249290599286304371, -58.00000000000012079 ) ) ;
#4738=AXIS2_PLACEMENT_3D ( 'NONE', #9923, #12294, #9707 ) ;
#4749=VECTOR ( 'NONE', #7283, 1000.000000000000000 ) ;
#4767=CARTESIAN_POINT ( 'NONE',  ( -0.9277479332649583021, -2.641590149077306826, -57.50000000000012079 ) ) ;
#4780=CARTESIAN_POINT ( 'NONE',  ( -20.99999999999998579, -2.249290599286303483, -38.00000000000012079 ) ) ;
#4781=CARTESIAN_POINT ( 'NONE',  ( -9.101643754575787781, 2.066879234150345024, -47.52815511422343775 ) ) ;
#4782=EDGE_CURVE ( 'NONE', #12049, #12792, #7193, .T. ) ;
#4783=DIRECTION ( 'NONE',  ( 1.000000000000000000, 0.000000000000000000, 0.000000000000000000 ) ) ;
#4789=SHAPE_REPRESENTATION_RELATIONSHIP ( 'NONE' , 'NONE' ,  #8914, #419 ) ;
#4791=CARTESIAN_POINT ( 'NONE',  ( -3.285520523750506516, 5.681530634152946568, -48.00000000000012079 ) ) ;
#4793=CARTESIAN_POINT ( 'NONE',  ( -8.982583014919022446, 1.839844381040865562, -48.00000000000012079 ) ) ;
#4794=EDGE_CURVE ( 'NONE', #12049, #11720, #4636, .T. ) ;
#4795=DIRECTION ( 'NONE',  ( 1.000000000000000000, 0.000000000000000000, 0.000000000000000000 ) ) ;
#4801=DIRECTION ( 'NONE',  ( -0.000000000000000000, 0.000000000000000000, 1.000000000000000000 ) ) ;
#4809=ADVANCED_FACE ( 'NONE', ( #9332 ), #7019, .F. ) ;
#4811=FACE_OUTER_BOUND ( 'NONE', #9991, .T. ) ;
#4824=DIRECTION ( 'NONE',  ( 0.8420378618367653223, 0.5394184268574524488, -0.000000000000000000 ) ) ;
#4828=CARTESIAN_POINT ( 'NONE',  ( -12.14523415828296571, -9.827631355817223024, -57.50000000000012079 ) ) ;
#4832=AXIS2_PLACEMENT_3D ( 'NONE', #14650, #12421, #3960 ) ;
#4838=CIRCLE ( 'NONE', #8070, 0.5000000000000008882 ) ;
#4841=CARTESIAN_POINT ( 'NONE',  ( -16.99999999999998579, -2.249290599286303927, -57.50000000000012079 ) ) ;
#4846=FACE_BOUND ( 'NONE', #7455, .T. ) ;
#4850=DIRECTION ( 'NONE',  ( 1.000000000000000000, 0.000000000000000000, 0.000000000000000000 ) ) ;
#4851=CARTESIAN_POINT ( 'NONE',  ( -8.982583014919022446, 1.839844381040865118, -47.50000000000012079 ) ) ;
#4854=ORIENTED_EDGE ( 'NONE', *, *, #6998, .T. ) ;
#4866=EDGE_CURVE ( 'NONE', #7624, #2373, #11117, .T. ) ;
#4877=VECTOR ( 'NONE', #10075, 1000.000000000000000 ) ;
#4887=FACE_OUTER_BOUND ( 'NONE', #6463, .T. ) ;
#4889=DIRECTION ( 'NONE',  ( -0.000000000000000000, -0.000000000000000000, 1.000000000000000000 ) ) ;
#4899=ORIENTED_EDGE ( 'NONE', *, *, #12571, .T. ) ;
#4900=CARTESIAN_POINT ( 'NONE',  ( -28.95977857253358323, -8.587818791446787614, -48.00000000000012079 ) ) ;
#4902=AXIS2_PLACEMENT_3D ( 'NONE', #3489, #4641, #14031 ) ;
#4906=EDGE_CURVE ( 'NONE', #490, #2898, #5799, .T. ) ;
#4919=ORIENTED_EDGE ( 'NONE', *, *, #386, .F. ) ;
#4921=DIRECTION ( 'NONE',  ( 0.000000000000000000, -1.000000000000000000, 0.000000000000000000 ) ) ;
#4924=AXIS2_PLACEMENT_3D ( 'NONE', #3935, #14707, #6265 ) ;
#4933=EDGE_CURVE ( 'NONE', #60, #6843, #6937, .T. ) ;
#4939=PRODUCT_CONTEXT ( 'NONE', #92, 'mechanical' ) ;
#4956=FACE_OUTER_BOUND ( 'NONE', #10380, .T. ) ;
#4959=DIRECTION ( 'NONE',  ( 1.000000000000000000, 0.000000000000000000, 0.000000000000000000 ) ) ;
#4971=AXIS2_PLACEMENT_3D ( 'NONE', #12092, #12163, #1620 ) ;
#4972=AXIS2_PLACEMENT_3D ( 'NONE', #119, #7113, #1340 ) ;
#4974=DIRECTION ( 'NONE',  ( 1.000000000000000000, 0.000000000000000000, 0.000000000000000000 ) ) ;
#4975=AXIS2_PLACEMENT_3D ( 'NONE', #15027, #7949, #9254 ) ;
#4976=VERTEX_POINT ( 'NONE', #4146 ) ;
#4980=CARTESIAN_POINT ( 'NONE',  ( -21.66581936427349575, -2.249290599286304371, -57.50000000000012079 ) ) ;
#4986=DIRECTION ( 'NONE',  ( -0.000000000000000000, -0.000000000000000000, 1.000000000000000000 ) ) ;
#4994=VERTEX_POINT ( 'NONE', #13466 ) ;
#4996=ORIENTED_EDGE ( 'NONE', *, *, #9151, .F. ) ;
#5001=CYLINDRICAL_SURFACE ( 'NONE', #4738, 0.4999999999999996114 ) ;
#5003=CIRCLE ( 'NONE', #13587, 3.694885682587998765 ) ;
#5023=CARTESIAN_POINT ( 'NONE',  ( -8.650962968042231083, 2.291620771759304898, -48.06291368403883268 ) ) ;
#5028=CARTESIAN_POINT ( 'NONE',  ( -9.345472082723105700, -7.632075232572700152, -48.02161282446750334 ) ) ;
#5031=CARTESIAN_POINT ( 'NONE',  ( -21.85476584171713199, 5.329050157244537900, 57.50000000000012079 ) ) ;
#5043=ORIENTED_EDGE ( 'NONE', *, *, #9837, .F. ) ;
#5046=VERTEX_POINT ( 'NONE', #8555 ) ;
#5048=ORIENTED_EDGE ( 'NONE', *, *, #5612, .F. ) ;
#5050=CARTESIAN_POINT ( 'NONE',  ( -9.345472082723105700, -7.632075232572700152, 48.02161282446750334 ) ) ;
#5066=ORIENTED_EDGE ( 'NONE', *, *, #1823, .F. ) ;
#5070=DIRECTION ( 'NONE',  ( 0.000000000000000000, -0.000000000000000000, -1.000000000000000000 ) ) ;
#5076=CIRCLE ( 'NONE', #9758, 0.5000000000000004441 ) ;
#5080=ORIENTED_EDGE ( 'NONE', *, *, #2292, .F. ) ;
#5081=CARTESIAN_POINT ( 'NONE',  ( -24.66543232906180805, 3.122884019241207287, 48.02064173568555816 ) ) ;
#5082=ADVANCED_FACE ( 'NONE', ( #9238 ), #6274, .F. ) ;
#5092=DIRECTION ( 'NONE',  ( -0.000000000000000000, 0.000000000000000000, 1.000000000000000000 ) ) ;
#5094=ORIENTED_EDGE ( 'NONE', *, *, #13338, .T. ) ;
#5096=AXIS2_PLACEMENT_3D ( 'NONE', #2661, #2585, #10742 ) ;
#5104=CARTESIAN_POINT ( 'NONE',  ( -8.679783256197868724, 2.339454207888506776, 48.10016682092218332 ) ) ;
#5112=CARTESIAN_POINT ( 'NONE',  ( -33.07225206673494711, -1.856991049495498425, 57.50000000000012079 ) ) ;
#5113=LINE ( 'NONE', #14276, #7916 ) ;
#5115=CARTESIAN_POINT ( 'NONE',  ( -24.80190065418678458, -6.760980545838084943, -48.43121057161747700 ) ) ;
#5129=DIRECTION ( 'NONE',  ( 0.000000000000000000, 0.000000000000000000, -1.000000000000000000 ) ) ;
#5134=ORIENTED_EDGE ( 'NONE', *, *, #12608, .F. ) ;
#5146=ORIENTED_EDGE ( 'NONE', *, *, #2957, .F. ) ;
#5149=DIRECTION ( 'NONE',  ( -0.5006040828730773384, 0.8656763553492754504, 0.000000000000000000 ) ) ;
#5151=B_SPLINE_CURVE_WITH_KNOTS ( 'NONE', 3,
 ( #4007, #11165, #8932, #6696, #2936, #13623, #5478, #11085, #10168, #7781 ),
 .UNSPECIFIED., .F., .F.,
 ( 4, 2, 2, 2, 4 ),
 ( 0.000000000000000000, 0.0003835113287520873016, 0.0007670226575041746032, 0.001150533986256262013, 0.001534045315008349206 ),
 .UNSPECIFIED. ) ;
#5153=EDGE_LOOP ( 'NONE', ( #603, #5509, #5997, #2264 ) ) ;
#5158=APPLICATION_CONTEXT ( 'automotive_design' ) ;
#5160=PLANE ( 'NONE',  #4971 ) ;
#5169=CARTESIAN_POINT ( 'NONE',  ( -5.290523468902621929, 4.522075770548486418, -57.50000000000012079 ) ) ;
#5172=ORIENTED_EDGE ( 'NONE', *, *, #7417, .T. ) ;
#5187=VECTOR ( 'NONE', #11066, 1000.000000000000114 ) ;
#5188=ORIENTED_EDGE ( 'NONE', *, *, #974, .T. ) ;
#5194=CIRCLE ( 'NONE', #2499, 0.4999999999999995559 ) ;
#5200=CARTESIAN_POINT ( 'NONE',  ( -21.16581936427349575, -2.249290599286304371, -50.50000000000012079 ) ) ;
#5207=AXIS2_PLACEMENT_3D ( 'NONE', #5707, #12626, #4384 ) ;
#5210=EDGE_LOOP ( 'NONE', ( #3817, #5925, #12985, #8662 ) ) ;
#5214=DIRECTION ( 'NONE',  ( 1.000000000000000000, 8.673617379884027583E-16, 0.000000000000000000 ) ) ;
#5239=DIRECTION ( 'NONE',  ( 1.000000000000000000, 0.000000000000000000, 0.000000000000000000 ) ) ;
#5245=EDGE_CURVE ( 'NONE', #10926, #981, #3289, .T. ) ;
#5249=AXIS2_PLACEMENT_3D ( 'NONE', #9246, #4701, #2391 ) ;
#5255=CARTESIAN_POINT ( 'NONE',  ( -9.209612907684750382, 2.258800220783480750, 47.62582736825572738 ) ) ;
#5256=ORIENTED_EDGE ( 'NONE', *, *, #12312, .T. ) ;
#5260=FACE_OUTER_BOUND ( 'NONE', #115, .T. ) ;
#5270=ORIENTED_EDGE ( 'NONE', *, *, #4866, .F. ) ;
#5272=DIRECTION ( 'NONE',  ( 1.000000000000000000, 0.000000000000000000, 0.000000000000000000 ) ) ;
#5279=DIRECTION ( 'NONE',  ( -0.8420378618367644341, -0.5394184268574535590, -0.000000000000000000 ) ) ;
#5291=CARTESIAN_POINT ( 'NONE',  ( -8.509932750408504276, 13.28409490805591808, 57.50000000000012079 ) ) ;
#5294=CARTESIAN_POINT ( 'NONE',  ( -12.83418063572647760, -2.249290599286303927, -50.00000000000012079 ) ) ;
#5295=ORIENTED_EDGE ( 'NONE', *, *, #12463, .T. ) ;
#5299=FACE_OUTER_BOUND ( 'NONE', #10332, .T. ) ;
#5305=EDGE_LOOP ( 'NONE', ( #683, #11068, #14117, #5938 ) ) ;
#5312=CARTESIAN_POINT ( 'NONE',  ( -10.08762850755046969, -8.023634329963208245, -47.66527511103321046 ) ) ;
#5314=ORIENTED_EDGE ( 'NONE', *, *, #503, .F. ) ;
#5315=CARTESIAN_POINT ( 'NONE',  ( -8.754378065084850391, 2.456381933588792865, -48.23869654929341522 ) ) ;
#5318=CARTESIAN_POINT ( 'NONE',  ( -16.99999999999998579, -2.249290599286303927, 58.00000000000012079 ) ) ;
#5331=CIRCLE ( 'NONE', #5096, 0.4999999999999999445 ) ;
#5333=AXIS2_PLACEMENT_3D ( 'NONE', #1343, #7037, #8503 ) ;
#5336=CARTESIAN_POINT ( 'NONE',  ( -24.96483633670257873, -6.441926561070030033, -48.01692658285762150 ) ) ;
#5337=ORIENTED_EDGE ( 'NONE', *, *, #4469, .F. ) ;
#5342=EDGE_LOOP ( 'NONE', ( #296, #12667 ) ) ;
#5346=EDGE_LOOP ( 'NONE', ( #13604, #961, #3865, #12162, #10595, #12330, #8973, #674, #2835, #8549, #9880 ) ) ;
#5347=DIRECTION ( 'NONE',  ( -0.000000000000000000, -0.000000000000000000, 1.000000000000000000 ) ) ;
#5355=TOROIDAL_SURFACE ( 'NONE', #12740, 8.500000000000000000, 0.5000000000000000000 ) ;
#5358=ADVANCED_FACE ( 'NONE', ( #9777 ), #5001, .T. ) ;
#5359=EDGE_LOOP ( 'NONE', ( #7356, #5636, #13280, #10495 ) ) ;
#5361=EDGE_LOOP ( 'NONE', ( #5066, #5956, #5919, #7313 ) ) ;
#5364=ORIENTED_EDGE ( 'NONE', *, *, #1789, .F. ) ;
#5365=CARTESIAN_POINT ( 'NONE',  ( -12.41494337171168283, -9.406612424898836977, -58.00000000000012079 ) ) ;
#5367=AXIS2_PLACEMENT_3D ( 'NONE', #3389, #2152, #7935 ) ;
#5368=DIRECTION ( 'NONE',  ( 1.000000000000000000, 0.000000000000000000, 0.000000000000000000 ) ) ;
#5372=ADVANCED_FACE ( 'NONE', ( #14390 ), #7196, .T. ) ;
#5373=DIRECTION ( 'NONE',  ( 0.000000000000000000, 0.000000000000000000, -1.000000000000000000 ) ) ;
#5375=DIRECTION ( 'NONE',  ( 0.000000000000000000, 0.000000000000000000, -1.000000000000000000 ) ) ;
#5377=CARTESIAN_POINT ( 'NONE',  ( -3.035218482312739496, 5.248692456477230373, 57.50000000000012079 ) ) ;
#5378=EDGE_CURVE ( 'NONE', #10204, #14789, #12632, .T. ) ;
#5381=CIRCLE ( 'NONE', #229, 0.5000000000000000000 ) ;
#5382=VERTEX_POINT ( 'NONE', #1606 ) ;
#5388=CARTESIAN_POINT ( 'NONE',  ( -24.38033816570045076, 2.914516366099690448, -47.90685900410169040 ) ) ;
#5389=CIRCLE ( 'NONE', #2929, 0.5000000000000000000 ) ;
#5390=CIRCLE ( 'NONE', #8096, 0.5000000000000004441 ) ;
#5393=CARTESIAN_POINT ( 'NONE',  ( -16.99999999999998579, -2.249290599286303927, 58.00000000000012079 ) ) ;
#5395=EDGE_CURVE ( 'NONE', #8222, #3759, #548, .T. ) ;
#5398=VERTEX_POINT ( 'NONE', #6444 ) ;
#5402=CARTESIAN_POINT ( 'NONE',  ( -9.097850607046364502, 2.059891325575069043, 47.52616914649232172 ) ) ;
#5408=ORIENTED_EDGE ( 'NONE', *, *, #4559, .F. ) ;
#5414=CARTESIAN_POINT ( 'NONE',  ( -24.80875755767168300, -6.748058119754043460, -48.36238429206898815 ) ) ;
#5418=DIRECTION ( 'NONE',  ( -0.8656763553492639041, -0.5006040828730973224, -0.000000000000000000 ) ) ;
#5420=VECTOR ( 'NONE', #11400, 1000.000000000000000 ) ;
#5421=EDGE_LOOP ( 'NONE', ( #12419, #9390, #7577, #1238 ) ) ;
#5426=EDGE_CURVE ( 'NONE', #11056, #12155, #6709, .T. ) ;
#5433=CARTESIAN_POINT ( 'NONE',  ( -25.24562193491511763, -6.954963132161501527, -48.23869654929341522 ) ) ;
#5435=DIRECTION ( 'NONE',  ( 1.224646799147353207E-16, 1.000000000000000000, -0.000000000000000000 ) ) ;
#5460=VERTEX_POINT ( 'NONE', #5294 ) ;
#5461=CARTESIAN_POINT ( 'NONE',  ( -30.80945343098651890, -5.389243620311580329, 48.00000000000012079 ) ) ;
#5472=CARTESIAN_POINT ( 'NONE',  ( -3.190546569013415379, 0.8906624217387615339, -48.50000000000012079 ) ) ;
#5477=DIRECTION ( 'NONE',  ( 0.000000000000000000, 0.000000000000000000, -1.000000000000000000 ) ) ;
#5478=CARTESIAN_POINT ( 'NONE',  ( -9.394882438906904554, 2.563636819302931524, 48.00656353678737531 ) ) ;
#5481=ORIENTED_EDGE ( 'NONE', *, *, #13730, .T. ) ;
#5484=EDGE_CURVE ( 'NONE', #4049, #7613, #4200, .T. ) ;
#5499=CARTESIAN_POINT ( 'NONE',  ( -24.64572710697934710, -6.998028550906933098, -47.88483805351501132 ) ) ;
#5501=ORIENTED_EDGE ( 'NONE', *, *, #11517, .F. ) ;
#5502=FACE_OUTER_BOUND ( 'NONE', #13366, .T. ) ;
#5507=VERTEX_POINT ( 'NONE', #9060 ) ;
#5509=ORIENTED_EDGE ( 'NONE', *, *, #13548, .T. ) ;
#5531=ORIENTED_EDGE ( 'NONE', *, *, #3488, .F. ) ;
#5537=DIRECTION ( 'NONE',  ( 0.000000000000000000, -1.000000000000000000, 0.000000000000000000 ) ) ;
#5542=DIRECTION ( 'NONE',  ( 1.000000000000000000, 3.565820478396769525E-15, 0.000000000000000000 ) ) ;
#5547=CARTESIAN_POINT ( 'NONE',  ( -12.14523415828296216, -9.827631355817223024, 57.50000000000012079 ) ) ;
#5554=EDGE_CURVE ( 'NONE', #7398, #3301, #6012, .T. ) ;
#5556=ORIENTED_EDGE ( 'NONE', *, *, #2468, .T. ) ;
#5559=AXIS2_PLACEMENT_3D ( 'NONE', #14865, #9256, #4478 ) ;
#5570=TOROIDAL_SURFACE ( 'NONE', #2109, 3.694885682587998765, 0.5000000000000000000 ) ;
#5574=ORIENTED_EDGE ( 'NONE', *, *, #12274, .F. ) ;
#5579=FACE_OUTER_BOUND ( 'NONE', #13006, .T. ) ;
#5599=CARTESIAN_POINT ( 'NONE',  ( -25.99999999999998934, -2.249290599286303927, 38.50000000000012790 ) ) ;
#5612=EDGE_CURVE ( 'NONE', #13646, #9532, #5996, .T. ) ;
#5613=CARTESIAN_POINT ( 'NONE',  ( -9.083879796419006780, -7.373836579503426414, 48.00000000000010658 ) ) ;
#5615=CIRCLE ( 'NONE', #2861, 4.194885682587998765 ) ;
#5635=FACE_OUTER_BOUND ( 'NONE', #9920, .T. ) ;
#5636=ORIENTED_EDGE ( 'NONE', *, *, #4315, .F. ) ;
#5639=LINE ( 'NONE', #14786, #14489 ) ;
#5640=CARTESIAN_POINT ( 'NONE',  ( -8.842479278987875446, -7.118053859731355182, -48.00000000000012079 ) ) ;
#5642=EDGE_LOOP ( 'NONE', ( #14165, #15, #10939, #8815 ) ) ;
#5650=EDGE_CURVE ( 'NONE', #14041, #2664, #5979, .T. ) ;
#5652=EDGE_LOOP ( 'NONE', ( #2393, #6011, #6291, #6234 ) ) ;
#5654=EDGE_LOOP ( 'NONE', ( #2573, #7902, #4682, #14784, #5364, #8634 ) ) ;
#5663=AXIS2_PLACEMENT_3D ( 'NONE', #3496, #4801, #14116 ) ;
#5668=DIRECTION ( 'NONE',  ( 0.8420378618367728718, 0.5394184268574404584, 0.000000000000000000 ) ) ;
#5669=LINE ( 'NONE', #9129, #6341 ) ;
#5670=CARTESIAN_POINT ( 'NONE',  ( -25.34493114703935035, -6.799303420495464323, -48.05421924268924272 ) ) ;
#5674=ORIENTED_EDGE ( 'NONE', *, *, #4718, .T. ) ;
#5677=DIRECTION ( 'NONE',  ( 1.000000000000000000, 0.000000000000000000, 0.000000000000000000 ) ) ;
#5692=AXIS2_PLACEMENT_3D ( 'NONE', #2772, #1831, #1613 ) ;
#5693=DIRECTION ( 'NONE',  ( 0.000000000000000000, 0.000000000000000000, -1.000000000000000000 ) ) ;
#5696=EDGE_CURVE ( 'NONE', #9532, #13060, #3672, .T. ) ;
#5698=ORIENTED_EDGE ( 'NONE', *, *, #12136, .T. ) ;
#5700=CARTESIAN_POINT ( 'NONE',  ( -7.999999999999986677, -2.249290599286302594, 47.50000000000012079 ) ) ;
#5703=CIRCLE ( 'NONE', #3966, 0.4999999999999997780 ) ;
#5707=CARTESIAN_POINT ( 'NONE',  ( -16.99999999999998579, -2.249290599286303927, -50.00000000000012079 ) ) ;
#5716=CIRCLE ( 'NONE', #6431, 9.500000000000001776 ) ;
#5717=CIRCLE ( 'NONE', #9898, 9.000000000000001776 ) ;
#5718=CARTESIAN_POINT ( 'NONE',  ( -8.563719136935748821, 2.126583234680710977, 48.00000000000012079 ) ) ;
#5726=CARTESIAN_POINT ( 'NONE',  ( -9.334567670938534789, -7.621465217813490511, -48.02064173568530236 ) ) ;
#5731=DIRECTION ( 'NONE',  ( -0.000000000000000000, -0.000000000000000000, 1.000000000000000000 ) ) ;
#5732=TOROIDAL_SURFACE ( 'NONE', #2239, 4.165819364273509962, 0.5000000000000000000 ) ;
#5734=DIRECTION ( 'NONE',  ( -0.8420378618367728718, -0.5394184268574404584, 0.000000000000000000 ) ) ;
#5739=ORIENTED_EDGE ( 'NONE', *, *, #214, .F. ) ;
#5741=B_SPLINE_CURVE_WITH_KNOTS ( 'NONE', 3,
 ( #13426, #12280, #3120, #8127, #14816, #6734, #9210, #12829 ),
 .UNSPECIFIED., .F., .F.,
 ( 4, 2, 2, 4 ),
 ( 5.291795217412410304E-17, 0.001077686929059509672, 0.002155373858118966434, 0.004310747716237871285 ),
 .UNSPECIFIED. ) ;
#5744=CARTESIAN_POINT ( 'NONE',  ( -8.787473001628837821, 2.499856724289235554, -48.50000000000012079 ) ) ;
#5749=CIRCLE ( 'NONE', #14817, 1.000000000000000888 ) ;
#5751=ADVANCED_FACE ( 'NONE', ( #14291 ), #3962, .F. ) ;
#5754=DIRECTION ( 'NONE',  ( 1.224646799147353207E-16, 1.000000000000000000, 0.000000000000000000 ) ) ;
#5755=CIRCLE ( 'NONE', #7213, 0.5000000000000004441 ) ;
#5757=DIRECTION ( 'NONE',  ( -0.000000000000000000, -0.000000000000000000, 1.000000000000000000 ) ) ;
#5771=EDGE_CURVE ( 'NONE', #12879, #7490, #3995, .T. ) ;
#5775=ORIENTED_EDGE ( 'NONE', *, *, #11997, .F. ) ;
#5776=DIRECTION ( 'NONE',  ( -0.8656763553492622387, -0.5006040828731004311, -0.000000000000000000 ) ) ;
#5779=EDGE_LOOP ( 'NONE', ( #9554, #5481, #8920, #2894 ) ) ;
#5783=DIRECTION ( 'NONE',  ( 0.000000000000000000, 0.000000000000000000, -1.000000000000000000 ) ) ;
#5784=CARTESIAN_POINT ( 'NONE',  ( -8.787473001628837821, 2.499856724289235554, 48.50000000000012079 ) ) ;
#5785=VERTEX_POINT ( 'NONE', #11046 ) ;
#5788=CARTESIAN_POINT ( 'NONE',  ( -24.54316048551696028, -7.158540021523408292, -48.50000000000012079 ) ) ;
#5791=ORIENTED_EDGE ( 'NONE', *, *, #4133, .F. ) ;
#5792=DIRECTION ( 'NONE',  ( 1.000000000000000000, 8.673617379884027583E-16, 0.000000000000000000 ) ) ;
#5798=FACE_OUTER_BOUND ( 'NONE', #12811, .T. ) ;
#5799=LINE ( 'NONE', #5882, #6447 ) ;
#5805=CARTESIAN_POINT ( 'NONE',  ( -9.271822474830662131, -6.861803161813125662, -47.50000000000012079 ) ) ;
#5807=EDGE_CURVE ( 'NONE', #12792, #505, #2593, .T. ) ;
#5809=VERTEX_POINT ( 'NONE', #4980 ) ;
#5810=AXIS2_PLACEMENT_3D ( 'NONE', #12391, #1769, #10009 ) ;
#5811=DIRECTION ( 'NONE',  ( 1.000000000000000000, 0.000000000000000000, 0.000000000000000000 ) ) ;
#5812=EDGE_LOOP ( 'NONE', ( #3888, #11324, #5739, #8717, #10690 ) ) ;
#5819=CIRCLE ( 'NONE', #14419, 4.194885682587998765 ) ;
#5834=ORIENTED_EDGE ( 'NONE', *, *, #284, .F. ) ;
#5839=ORIENTED_EDGE ( 'NONE', *, *, #5245, .T. ) ;
#5842=AXIS2_PLACEMENT_3D ( 'NONE', #6307, #14469, #5149 ) ;
#5843=TOROIDAL_SURFACE ( 'NONE', #14441, 8.500000000000000000, 0.5000000000000000000 ) ;
#5847=CARTESIAN_POINT ( 'NONE',  ( -9.619661834299611414, -7.413097564672328055, 47.90685900409895481 ) ) ;
#5848=ORIENTED_EDGE ( 'NONE', *, *, #5916, .F. ) ;
#5858=EDGE_CURVE ( 'NONE', #14041, #5809, #2543, .T. ) ;
#5868=EDGE_CURVE ( 'NONE', #8531, #3355, #3518, .T. ) ;
#5875=ORIENTED_EDGE ( 'NONE', *, *, #3201, .F. ) ;
#5877=ORIENTED_EDGE ( 'NONE', *, *, #5868, .F. ) ;
#5879=DIRECTION ( 'NONE',  ( 1.000000000000000000, 0.000000000000000000, 0.000000000000000000 ) ) ;
#5880=B_SPLINE_CURVE_WITH_KNOTS ( 'NONE', 3,
 ( #8628, #11302, #5315, #14699, #4151, #7704 ),
 .UNSPECIFIED., .F., .F.,
 ( 4, 2, 4 ),
 ( 0.000000000000000000, 0.0003908577252344195446, 0.0007817154504688390891 ),
 .UNSPECIFIED. ) ;
#5882=CARTESIAN_POINT ( 'NONE',  ( -20.99999999999998579, -2.249290599286303483, -47.31370849898487307 ) ) ;
#5884=DIRECTION ( 'NONE',  ( -0.8420378618367728718, -0.5394184268574404584, -0.000000000000000000 ) ) ;
#5889=CYLINDRICAL_SURFACE ( 'NONE', #964, 0.5000000000000000000 ) ;
#5893=ORIENTED_EDGE ( 'NONE', *, *, #15185, .T. ) ;
#5897=DIRECTION ( 'NONE',  ( -1.000000000000000000, 0.000000000000000000, 0.000000000000000000 ) ) ;
#5900=AXIS2_PLACEMENT_3D ( 'NONE', #6538, #7780, #4389 ) ;
#5910=ORIENTED_EDGE ( 'NONE', *, *, #9078, .T. ) ;
#5916=EDGE_CURVE ( 'NONE', #12879, #5460, #3750, .T. ) ;
#5919=ORIENTED_EDGE ( 'NONE', *, *, #13830, .F. ) ;
#5925=ORIENTED_EDGE ( 'NONE', *, *, #10744, .F. ) ;
#5931=CARTESIAN_POINT ( 'NONE',  ( -23.68126483017411488, 3.790603994468874749, -47.74939190649463683 ) ) ;
#5938=ORIENTED_EDGE ( 'NONE', *, *, #13409, .T. ) ;
#5945=EDGE_CURVE ( 'NONE', #14442, #2373, #12674, .T. ) ;
#5950=LINE ( 'NONE', #9569, #3098 ) ;
#5953=VECTOR ( 'NONE', #5279, 1000.000000000000000 ) ;
#5955=CARTESIAN_POINT ( 'NONE',  ( -33.07225206673494711, -1.856991049495498425, 48.00000000000012079 ) ) ;
#5956=ORIENTED_EDGE ( 'NONE', *, *, #3727, .T. ) ;
#5957=CARTESIAN_POINT ( 'NONE',  ( -8.679783256197868724, 2.339454207888506776, -48.10016682092218332 ) ) ;
#5964=CARTESIAN_POINT ( 'NONE',  ( -16.99999999999998579, -2.249290599286303927, 58.00000000000012079 ) ) ;
#5979=CIRCLE ( 'NONE', #14560, 5.165819364273509073 ) ;
#5981=CARTESIAN_POINT ( 'NONE',  ( -25.01741698508091005, -6.338425579613558014, 47.50000000000012079 ) ) ;
#5989=AXIS2_PLACEMENT_3D ( 'NONE', #9759, #14445, #3892 ) ;
#5993=ORIENTED_EDGE ( 'NONE', *, *, #14627, .T. ) ;
#5996=LINE ( 'NONE', #8373, #3986 ) ;
#5997=ORIENTED_EDGE ( 'NONE', *, *, #9565, .F. ) ;
#5999=CARTESIAN_POINT ( 'NONE',  ( -32.80254285330629216, -2.278009980413787439, 57.50000000000012079 ) ) ;
#6005=LINE ( 'NONE', #3823, #904 ) ;
#6009=EDGE_LOOP ( 'NONE', ( #14756, #14959, #6945, #498, #511, #9502, #6783, #1450, #1469, #12895 ) ) ;
#6011=ORIENTED_EDGE ( 'NONE', *, *, #1928, .F. ) ;
#6012=CIRCLE ( 'NONE', #7965, 1.000000000000000888 ) ;
#6021=DIRECTION ( 'NONE',  ( 1.000000000000000000, 0.000000000000000000, 0.000000000000000000 ) ) ;
#6023=CARTESIAN_POINT ( 'NONE',  ( -24.91612020358099855, 2.875255380930533455, 48.00000000000010658 ) ) ;
#6026=CARTESIAN_POINT ( 'NONE',  ( -3.190546569013415379, 0.8906624217387615339, -57.50000000000012079 ) ) ;
#6028=DIRECTION ( 'NONE',  ( 0.000000000000000000, 0.000000000000000000, 1.000000000000000000 ) ) ;
#6029=DIRECTION ( 'NONE',  ( 1.000000000000000000, -1.214306433183763862E-14, 0.000000000000000000 ) ) ;
#6030=ORIENTED_EDGE ( 'NONE', *, *, #11161, .T. ) ;
#6031=CARTESIAN_POINT ( 'NONE',  ( -9.263396839842437558, 2.349907881949450772, -47.70033363922482295 ) ) ;
#6036=EDGE_CURVE ( 'NONE', #4463, #3566, #5151, .T. ) ;
#6038=ORIENTED_EDGE ( 'NONE', *, *, #7880, .T. ) ;
#6045=EDGE_CURVE ( 'NONE', #2221, #5382, #9948, .T. ) ;
#6050=CARTESIAN_POINT ( 'NONE',  ( -25.24934951899391322, -6.946659123520668722, 48.24789848114230040 ) ) ;
#6051=CIRCLE ( 'NONE', #1854, 8.500000000000000000 ) ;
#6058=VERTEX_POINT ( 'NONE', #5169 ) ;
#6070=ORIENTED_EDGE ( 'NONE', *, *, #1124, .F. ) ;
#6074=VERTEX_POINT ( 'NONE', #14622 ) ;
#6078=AXIS2_PLACEMENT_3D ( 'NONE', #9461, #1291, #3680 ) ;
#6084=DIRECTION ( 'NONE',  ( -0.000000000000000000, 0.000000000000000000, 1.000000000000000000 ) ) ;
#6097=ADVANCED_FACE ( 'NONE', ( #12472 ), #8773, .T. ) ;
#6101=DIRECTION ( 'NONE',  ( 1.000000000000000000, 0.000000000000000000, 0.000000000000000000 ) ) ;
#6104=DIRECTION ( 'NONE',  ( -0.8420378618367653223, -0.5394184268574524488, -0.000000000000000000 ) ) ;
#6107=CARTESIAN_POINT ( 'NONE',  ( -8.750650481006019277, 2.448077924947977380, -48.24789848114231461 ) ) ;
#6109=AXIS2_PLACEMENT_3D ( 'NONE', #12054, #217, #9761 ) ;
#6128=DIRECTION ( 'NONE',  ( -0.5125013958363011657, -0.8586863916854879930, -0.000000000000000000 ) ) ;
#6133=ADVANCED_FACE ( 'NONE', ( #8249 ), #10662, .T. ) ;
#6155=DIRECTION ( 'NONE',  ( 1.000000000000000000, 8.270659117969274159E-16, 0.000000000000000000 ) ) ;
#6162=CARTESIAN_POINT ( 'NONE',  ( -11.45041300328984413, -9.336677115435668028, 48.21133583021728697 ) ) ;
#6164=AXIS2_PLACEMENT_3D ( 'NONE', #887, #3285, #9057 ) ;
#6166=CARTESIAN_POINT ( 'NONE',  ( -21.66581936427349575, -2.249290599286303483, 50.50000000000012079 ) ) ;
#6170=DIRECTION ( 'NONE',  ( 1.000000000000000000, 1.789942591005740441E-15, 0.000000000000000000 ) ) ;
#6171=EDGE_CURVE ( 'NONE', #7961, #4611, #9434, .T. ) ;
#6174=AXIS2_PLACEMENT_3D ( 'NONE', #1796, #1936, #6489 ) ;
#6175=EDGE_CURVE ( 'NONE', #10987, #7187, #6769, .T. ) ;
#6185=CARTESIAN_POINT ( 'NONE',  ( -8.563719136935748821, 2.126583234680710977, -48.00000000000012079 ) ) ;
#6192=CIRCLE ( 'NONE', #9121, 4.000000000000000000 ) ;
#6201=CARTESIAN_POINT ( 'NONE',  ( -24.54316048551696028, -7.158540021523408292, -48.50000000000012079 ) ) ;
#6206=TOROIDAL_SURFACE ( 'NONE', #9885, 1.000000000000000000, 0.5000000000000000000 ) ;
#6225=EDGE_CURVE ( 'NONE', #15020, #56, #336, .T. ) ;
#6226=DIRECTION ( 'NONE',  ( -0.4543483311474731945, 0.8908241094534353754, 0.000000000000000000 ) ) ;
#6232=ORIENTED_EDGE ( 'NONE', *, *, #7752, .T. ) ;
#6234=ORIENTED_EDGE ( 'NONE', *, *, #2568, .F. ) ;
#6235=CARTESIAN_POINT ( 'NONE',  ( -24.96222495693456978, -7.431276100536581275, -57.50000000000012079 ) ) ;
#6243=AXIS2_PLACEMENT_3D ( 'NONE', #7312, #1544, #6021 ) ;
#6245=EDGE_CURVE ( 'NONE', #3062, #10926, #5003, .T. ) ;
#6259=DIRECTION ( 'NONE',  ( 1.000000000000000000, 0.000000000000000000, 0.000000000000000000 ) ) ;
#6261=CARTESIAN_POINT ( 'NONE',  ( -11.54807159409575235, -9.445082653969818054, -48.38495513067856280 ) ) ;
#6265=DIRECTION ( 'NONE',  ( 1.000000000000000000, 0.000000000000000000, 0.000000000000000000 ) ) ;
#6267=DIRECTION ( 'NONE',  ( 1.000000000000000000, 0.000000000000000000, 0.000000000000000000 ) ) ;
#6274=( BOUNDED_SURFACE ( )  B_SPLINE_SURFACE ( 3, 2, ( 
 ( #12693, #6841, #13696 ),
 ( #1989, #10392, #10161 ),
 ( #681, #5388, #8924 ),
 ( #10084, #14846, #10231 ),
 ( #1840, #11527, #2147 ),
 ( #8996, #3152, #13618 ),
 ( #7852, #14922, #11299 ),
 ( #1916, #10310, #912 ) ),
 .UNSPECIFIED., .F., .F., .F. ) 
 B_SPLINE_SURFACE_WITH_KNOTS ( ( 4, 2, 2, 4 ),
 ( 3, 3 ),
 ( 0.000000000000000000, 0.001129222206655581574, 0.002258444413311163149, 0.004516888826622326297 ),
 ( 0.000000000000000000, 1.000000000000000000 ),
 .UNSPECIFIED. ) 
 GEOMETRIC_REPRESENTATION_ITEM ( )  RATIONAL_B_SPLINE_SURFACE ( (
 ( 1.000000000000000000, 0.7071067811864936159, 1.000000000000000000),
 ( 1.000000000000000000, 0.7608707698420138499, 1.000000000000000000),
 ( 1.000000000000000000, 0.8047257278452277784, 1.000000000000000000),
 ( 1.000000000000000000, 0.8783509392183566078, 1.000000000000000000),
 ( 1.000000000000000000, 0.9081758943102266057, 1.000000000000000000),
 ( 1.000000000000000000, 0.9781389570711758186, 1.000000000000000000),
 ( 1.000000000000000000, 0.9996704379314563793, 1.000000000000000000),
 ( 1.000000000000000000, 1.000000000000000000, 1.000000000000000000) ) ) 
 REPRESENTATION_ITEM ( '' )  SURFACE ( )  );
#6275=FACE_OUTER_BOUND ( 'NONE', #727, .T. ) ;
#6278=ORIENTED_EDGE ( 'NONE', *, *, #13891, .F. ) ;
#6282=CYLINDRICAL_SURFACE ( 'NONE', #1282, 4.000000000000000000 ) ;
#6283=CARTESIAN_POINT ( 'NONE',  ( -12.83418063572647760, -2.249290599286303927, -50.50000000000012079 ) ) ;
#6291=ORIENTED_EDGE ( 'NONE', *, *, #641, .F. ) ;
#6293=VERTEX_POINT ( 'NONE', #8401 ) ;
#6298=EDGE_CURVE ( 'NONE', #7044, #4976, #5749, .T. ) ;
#6299=ORIENTED_EDGE ( 'NONE', *, *, #6245, .T. ) ;
#6301=DIRECTION ( 'NONE',  ( 0.8656763553492622387, 0.5006040828731004311, -0.000000000000000000 ) ) ;
#6304=ORIENTED_EDGE ( 'NONE', *, *, #2037, .F. ) ;
#6305=AXIS2_PLACEMENT_3D ( 'NONE', #1915, #4294, #12460 ) ;
#6307=CARTESIAN_POINT ( 'NONE',  ( -28.95977857253363297, -8.587818791446675704, -48.50000000000012079 ) ) ;
#6315=AXIS2_PLACEMENT_3D ( 'NONE', #4082, #8567, #11096 ) ;
#6316=ADVANCED_FACE ( 'NONE', ( #8480 ), #11887, .T. ) ;
#6320=AXIS2_PLACEMENT_3D ( 'NONE', #10213, #14985, #5368 ) ;
#6326=CARTESIAN_POINT ( 'NONE',  ( -9.457494889590920550, -7.172893779636416056, -47.50000000000009237 ) ) ;
#6331=CARTESIAN_POINT ( 'NONE',  ( -16.99999999999998579, -2.249290599286303927, 57.50000000000012079 ) ) ;
#6334=CARTESIAN_POINT ( 'NONE',  ( -9.456839502978525047, 2.659958805273927140, 48.36906329404666849 ) ) ;
#6341=VECTOR ( 'NONE', #10436, 1000.000000000000000 ) ;
#6344=FACE_OUTER_BOUND ( 'NONE', #1253, .T. ) ;
#6348=ORIENTED_EDGE ( 'NONE', *, *, #13363, .F. ) ;
#6349=DIRECTION ( 'NONE',  ( -0.000000000000000000, -0.000000000000000000, 1.000000000000000000 ) ) ;
#6352=DIRECTION ( 'NONE',  ( 1.000000000000000000, 0.000000000000000000, 0.000000000000000000 ) ) ;
#6353=ORIENTED_EDGE ( 'NONE', *, *, #11242, .F. ) ;
#6357=EDGE_CURVE ( 'NONE', #12008, #7657, #2695, .T. ) ;
#6358=EDGE_CURVE ( 'NONE', #13865, #2105, #8921, .T. ) ;
#6360=CARTESIAN_POINT ( 'NONE',  ( 0.5043391135745837195, 0.8906624217387615339, 58.00000000000012079 ) ) ;
#6365=ORIENTED_EDGE ( 'NONE', *, *, #2058, .F. ) ;
#6366=CARTESIAN_POINT ( 'NONE',  ( -23.68126483017411488, 3.790603994468874749, 47.74939190649463683 ) ) ;
#6370=EDGE_CURVE ( 'NONE', #11451, #13978, #12124, .T. ) ;
#6376=VERTEX_POINT ( 'NONE', #14323 ) ;
#6381=FACE_OUTER_BOUND ( 'NONE', #5359, .T. ) ;
#6385=ORIENTED_EDGE ( 'NONE', *, *, #6585, .T. ) ;
#6394=CARTESIAN_POINT ( 'NONE',  ( -8.537170960192327129, 2.067018546614582508, -58.00000000000012079 ) ) ;
#6397=CARTESIAN_POINT ( 'NONE',  ( -9.456839514482961562, 2.659958822950721835, 48.50000000000012079 ) ) ;
#6403=TOROIDAL_SURFACE ( 'NONE', #13052, 4.165819364273509962, 0.5000000000000000000 ) ;
#6407=CARTESIAN_POINT ( 'NONE',  ( -24.12409601409935078, -6.885803942510236197, 57.50000000000012079 ) ) ;
#6408=EDGE_CURVE ( 'NONE', #5046, #10853, #1802, .T. ) ;
#6414=AXIS2_PLACEMENT_3D ( 'NONE', #7310, #8248, #2389 ) ;
#6422=DIRECTION ( 'NONE',  ( 1.000000000000000000, 0.000000000000000000, 0.000000000000000000 ) ) ;
#6423=EDGE_LOOP ( 'NONE', ( #5501, #15086, #11912, #9333 ) ) ;
#6425=AXIS2_PLACEMENT_3D ( 'NONE', #1458, #9312, #7003 ) ;
#6426=AXIS2_PLACEMENT_3D ( 'NONE', #4406, #9110, #3258 ) ;
#6431=AXIS2_PLACEMENT_3D ( 'NONE', #2962, #4176, #5272 ) ;
#6444=CARTESIAN_POINT ( 'NONE',  ( -5.290523468902621929, 4.522075770548486418, -48.50000000000012079 ) ) ;
#6446=CIRCLE ( 'NONE', #7645, 0.5000000000000000000 ) ;
#6447=VECTOR ( 'NONE', #10567, 1000.000000000000000 ) ;
#6452=DIRECTION ( 'NONE',  ( 1.000000000000000000, 0.000000000000000000, 0.000000000000000000 ) ) ;
#6453=DIRECTION ( 'NONE',  ( 1.000000000000000000, 0.000000000000000000, 0.000000000000000000 ) ) ;
#6458=VECTOR ( 'NONE', #7811, 1000.000000000000000 ) ;
#6463=EDGE_LOOP ( 'NONE', ( #5791, #4854, #11443, #13783 ) ) ;
#6480=CARTESIAN_POINT ( 'NONE',  ( -8.750650481006019277, 2.448077924947977380, 48.24789848114231461 ) ) ;
#6489=DIRECTION ( 'NONE',  ( 0.8420378618367644341, 0.5394184268574535590, 0.000000000000000000 ) ) ;
#6490=CARTESIAN_POINT ( 'NONE',  ( -25.01741698508091005, -6.338425579613558014, -47.50000000000012079 ) ) ;
#6495=CARTESIAN_POINT ( 'NONE',  ( -21.66581936427349575, -2.249290599286303483, 50.00000000000012079 ) ) ;
#6497=ADVANCED_FACE ( 'NONE', ( #8686 ), #4056, .T. ) ;
#6498=ORIENTED_EDGE ( 'NONE', *, *, #2503, .F. ) ;
#6512=CARTESIAN_POINT ( 'NONE',  ( -9.037775043065350289, 2.932694901963889933, -48.50000000000012079 ) ) ;
#6516=ADVANCED_FACE ( 'NONE', ( #6381 ), #744, .T. ) ;
#6519=DIRECTION ( 'NONE',  ( 0.000000000000000000, -1.000000000000000000, 0.000000000000000000 ) ) ;
#6523=AXIS2_PLACEMENT_3D ( 'NONE', #8789, #13484, #12334 ) ;
#6524=CARTESIAN_POINT ( 'NONE',  ( -16.99999999999998579, -2.249290599286303927, 58.00000000000012079 ) ) ;
#6538=CARTESIAN_POINT ( 'NONE',  ( -16.99999999999998579, -2.249290599286303927, 50.00000000000012079 ) ) ;
#6541=DIRECTION ( 'NONE',  ( -0.5006040828730242698, 0.8656763553493063146, 0.000000000000000000 ) ) ;
#6549=ADVANCED_FACE ( 'NONE', ( #9997 ), #953, .F. ) ;
#6550=CARTESIAN_POINT ( 'NONE',  ( -16.99999999999998579, -2.249290599286303927, 57.50000000000012079 ) ) ;
#6551=ORIENTED_EDGE ( 'NONE', *, *, #6245, .F. ) ;
#6552=AXIS2_PLACEMENT_3D ( 'NONE', #903, #5537, #5693 ) ;
#6557=LINE ( 'NONE', #13722, #10563 ) ;
#6560=ORIENTED_EDGE ( 'NONE', *, *, #8948, .F. ) ;
#6580=DIRECTION ( 'NONE',  ( -0.000000000000000000, 1.000000000000000000, 0.000000000000000000 ) ) ;
#6583=DIRECTION ( 'NONE',  ( -1.000000000000000000, 0.000000000000000000, 0.000000000000000000 ) ) ;
#6585=EDGE_CURVE ( 'NONE', #12155, #298, #12853, .T. ) ;
#6615=ORIENTED_EDGE ( 'NONE', *, *, #6171, .T. ) ;
#6617=CARTESIAN_POINT ( 'NONE',  ( -25.04138923958014473, -6.321889167469157300, 58.00000000000012079 ) ) ;
#6625=CARTESIAN_POINT ( 'NONE',  ( -9.038486528834313916, 1.949452350488303454, 47.50000000626571506 ) ) ;
#6627=CARTESIAN_POINT ( 'NONE',  ( -28.95977857253349796, -8.587818791446737876, -48.50000000000012079 ) ) ;
#6636=CARTESIAN_POINT ( 'NONE',  ( -24.90214939295363550, -6.558472524147630267, -47.52616914649232172 ) ) ;
#6637=ADVANCED_FACE ( 'NONE', ( #14149 ), #10685, .T. ) ;
#6652=DIRECTION ( 'NONE',  ( 0.000000000000000000, -0.000000000000000000, -1.000000000000000000 ) ) ;
#6654=DIRECTION ( 'NONE',  ( 0.000000000000000000, 0.000000000000000000, -1.000000000000000000 ) ) ;
#6658=EDGE_LOOP ( 'NONE', ( #15134, #5775, #2998, #11011 ) ) ;
#6666=EDGE_CURVE ( 'NONE', #10292, #355, #1366, .T. ) ;
#6667=CARTESIAN_POINT ( 'NONE',  ( 0.000000000000000000, 0.000000000000000000, -58.00000000000012079 ) ) ;
#6669=ORIENTED_EDGE ( 'NONE', *, *, #6298, .F. ) ;
#6671=EDGE_CURVE ( 'NONE', #10590, #15020, #2528, .T. ) ;
#6680=DIRECTION ( 'NONE',  ( 0.000000000000000000, 0.000000000000000000, 1.000000000000000000 ) ) ;
#6684=AXIS2_PLACEMENT_3D ( 'NONE', #5461, #6680, #3147 ) ;
#6691=CARTESIAN_POINT ( 'NONE',  ( -5.040221427466109461, 4.089237592873833371, -58.00000000000012079 ) ) ;
#6696=CARTESIAN_POINT ( 'NONE',  ( -9.215065577852303846, 2.268247386559545387, 47.63220435834860922 ) ) ;
#6700=AXIS2_PLACEMENT_3D ( 'NONE', #6331, #11024, #8630 ) ;
#6708=PRODUCT_DEFINITION_SHAPE ( 'NONE', 'NONE',  #7585 ) ;
#6709=B_SPLINE_CURVE_WITH_KNOTS ( 'NONE', 3,
 ( #14600, #3762, #593, #9626, #8472, #13157, #1455, #6162, #7382, #12074, #3061, #12604 ),
 .UNSPECIFIED., .F., .F.,
 ( 4, 2, 2, 2, 2, 4 ),
 ( 0.000000000000000000, 0.001071381053236907443, 0.002142762106473816621, 0.003214143159710726016, 0.003749833686329184183, 0.004285524212947642783 ),
 .UNSPECIFIED. ) ;
#6714=CYLINDRICAL_SURFACE ( 'NONE', #451, 0.5000000000000000000 ) ;
#6716=DIRECTION ( 'NONE',  ( 1.000000000000000000, 0.000000000000000000, 0.000000000000000000 ) ) ;
#6726=CARTESIAN_POINT ( 'NONE',  ( -22.16581936427349575, -2.249290599286303483, 58.00000000000012079 ) ) ;
#6734=CARTESIAN_POINT ( 'NONE',  ( -23.02941217286474185, 4.529839663208023559, -48.26891069786830002 ) ) ;
#6736=CARTESIAN_POINT ( 'NONE',  ( -12.33418063572647938, -2.249290599286303927, 50.50000000000012079 ) ) ;
#6749=CARTESIAN_POINT ( 'NONE',  ( 1.004339113574583608, 0.8906624217387615339, 48.50000000000012079 ) ) ;
#6751=( BOUNDED_SURFACE ( )  B_SPLINE_SURFACE ( 3, 2, ( 
 ( #10257, #14951, #2091 ),
 ( #933, #3786, #14108 ),
 ( #8492, #329, #10715 ),
 ( #6107, #14339, #13175 ),
 ( #3851, #9651, #2564 ),
 ( #5957, #9575, #6031 ),
 ( #5023, #2631, #1399 ),
 ( #8556, #10642, #175 ),
 ( #6185, #7021, #107 ),
 ( #7102, #4793, #7325 ) ),
 .UNSPECIFIED., .F., .F., .F. ) 
 B_SPLINE_SURFACE_WITH_KNOTS ( ( 4, 2, 2, 2, 4 ),
 ( 3, 3 ),
 ( 0.0006711510808134562266, 0.001062132081067026709, 0.001453113081320596975, 0.001844094081574167241, 0.002235075081827737724 ),
 ( 0.000000000000000000, 1.000000000000000000 ),
 .UNSPECIFIED. ) 
 GEOMETRIC_REPRESENTATION_ITEM ( )  RATIONAL_B_SPLINE_SURFACE ( (
 ( 1.000000000000000000, 0.7254762501100212591, 1.000000000000000000),
 ( 1.000000000000000000, 0.7255094664176575670, 1.000000000000000000),
 ( 1.000000000000000000, 0.7239949553645330660, 1.000000000000000000),
 ( 1.000000000000000000, 0.7190573720639517052, 1.000000000000000000),
 ( 1.000000000000000000, 0.7156412189950384084, 1.000000000000000000),
 ( 1.000000000000000000, 0.7094102539595253942, 1.000000000000000000),
 ( 1.000000000000000000, 0.7066203625162220670, 1.000000000000000000),
 ( 1.000000000000000000, 0.7042417591948760824, 1.000000000000000000),
 ( 1.000000000000000000, 0.7046402682200600953, 1.000000000000000000),
 ( 1.000000000000000000, 0.7071067811865475727, 1.000000000000000000) ) ) 
 REPRESENTATION_ITEM ( '' )  SURFACE ( )  );
#6758=ORIENTED_EDGE ( 'NONE', *, *, #9567, .T. ) ;
#6762=EDGE_CURVE ( 'NONE', #7744, #922, #2371, .T. ) ;
#6769=LINE ( 'NONE', #10239, #1057 ) ;
#6779=ADVANCED_FACE ( 'NONE', ( #8232 ), #2447, .T. ) ;
#6783=ORIENTED_EDGE ( 'NONE', *, *, #8202, .T. ) ;
#6801=VERTEX_POINT ( 'NONE', #4115 ) ;
#6804=AXIS2_PLACEMENT_3D ( 'NONE', #4275, #8976, #4127 ) ;
#6809=DIRECTION ( 'NONE',  ( -1.000000000000000000, 0.000000000000000000, 0.000000000000000000 ) ) ;
#6818=DIRECTION ( 'NONE',  ( 1.000000000000000000, 0.000000000000000000, 0.000000000000000000 ) ) ;
#6821=AXIS2_PLACEMENT_3D ( 'NONE', #7976, #5757, #13977 ) ;
#6827=FACE_OUTER_BOUND ( 'NONE', #5361, .T. ) ;
#6830=CARTESIAN_POINT ( 'NONE',  ( -10.96079405803985729, -9.021238043844263643, 48.26696389624903816 ) ) ;
#6834=DIRECTION ( 'NONE',  ( -0.000000000000000000, 0.000000000000000000, 1.000000000000000000 ) ) ;
#6841=CARTESIAN_POINT ( 'NONE',  ( -24.72817752516935741, 2.363221963240438761, -48.00000000000019185 ) ) ;
#6843=VERTEX_POINT ( 'NONE', #7667 ) ;
#6856=CIRCLE ( 'NONE', #5900, 4.165819364273509962 ) ;
#6860=CARTESIAN_POINT ( 'NONE',  ( -9.037775043065352065, 2.932694901963889489, 57.50000000000012079 ) ) ;
#6867=FACE_OUTER_BOUND ( 'NONE', #915, .T. ) ;
#6868=EDGE_CURVE ( 'NONE', #13646, #7307, #14736, .T. ) ;
#6886=CARTESIAN_POINT ( 'NONE',  ( -16.99999999999998579, -2.249290599286303927, 47.50000000000012079 ) ) ;
#6887=DIRECTION ( 'NONE',  ( 1.000000000000000000, 0.000000000000000000, 0.000000000000000000 ) ) ;
#6905=DIRECTION ( 'NONE',  ( 1.000000000000000000, 0.000000000000000000, 0.000000000000000000 ) ) ;
#6911=AXIS2_PLACEMENT_3D ( 'NONE', #12961, #10494, #15190 ) ;
#6913=CIRCLE ( 'NONE', #13542, 0.5000000000000004441 ) ;
#6914=DIRECTION ( 'NONE',  ( 1.000000000000000000, 0.000000000000000000, 0.000000000000000000 ) ) ;
#6920=CARTESIAN_POINT ( 'NONE',  ( -22.94555154978778688, 4.515786682032536525, -48.04486892757390848 ) ) ;
#6924=CARTESIAN_POINT ( 'NONE',  ( -8.537170960192302260, 2.067018546614596719, 47.50000000000012079 ) ) ;
#6937=CIRCLE ( 'NONE', #781, 4.665819364273509073 ) ;
#6940=DIRECTION ( 'NONE',  ( -0.000000000000000000, 0.000000000000000000, 1.000000000000000000 ) ) ;
#6941=ORIENTED_EDGE ( 'NONE', *, *, #12136, .F. ) ;
#6943=FACE_OUTER_BOUND ( 'NONE', #13609, .T. ) ;
#6945=ORIENTED_EDGE ( 'NONE', *, *, #12274, .T. ) ;
#6948=CIRCLE ( 'NONE', #11353, 0.5000000000000004441 ) ;
#6952=CARTESIAN_POINT ( 'NONE',  ( -8.842479278987921631, -7.118053859731281463, -48.00000000000012079 ) ) ;
#6954=DIRECTION ( 'NONE',  ( 0.000000000000000000, 0.000000000000000000, -1.000000000000000000 ) ) ;
#6956=ORIENTED_EDGE ( 'NONE', *, *, #8609, .T. ) ;
#6963=DIRECTION ( 'NONE',  ( 0.5006040828730989878, -0.8656763553492631269, 0.000000000000000000 ) ) ;
#6969=CARTESIAN_POINT ( 'NONE',  ( -16.99999999999998579, -2.249290599286303927, -47.50000000000012079 ) ) ;
#6974=EDGE_CURVE ( 'NONE', #8990, #10346, #5741, .T. ) ;
#6991=CARTESIAN_POINT ( 'NONE',  ( -12.14523415828296216, -9.827631355817223024, 48.00000000000012079 ) ) ;
#6996=DIRECTION ( 'NONE',  ( -0.8420378618367728718, -0.5394184268574404584, -0.000000000000000000 ) ) ;
#6998=EDGE_CURVE ( 'NONE', #6293, #11451, #1170, .T. ) ;
#7002=ORIENTED_EDGE ( 'NONE', *, *, #2638, .F. ) ;
#7003=DIRECTION ( 'NONE',  ( -0.8656763553492639041, -0.5006040828730973224, 0.000000000000000000 ) ) ;
#7012=EDGE_CURVE ( 'NONE', #3688, #4595, #9417, .T. ) ;
#7019=PLANE ( 'NONE',  #2015 ) ;
#7020=VERTEX_POINT ( 'NONE', #3350 ) ;
#7021=CARTESIAN_POINT ( 'NONE',  ( -9.009135308666337494, 1.891904487837172688, -48.00342231809197102 ) ) ;
#7023=DIRECTION ( 'NONE',  ( 1.000000000000000000, 0.000000000000000000, 0.000000000000000000 ) ) ;
#7037=DIRECTION ( 'NONE',  ( 0.8656763553493069807, 0.5006040828730229375, -0.000000000000000000 ) ) ;
#7038=DIRECTION ( 'NONE',  ( 0.000000000000000000, 0.000000000000000000, 1.000000000000000000 ) ) ;
#7041=CARTESIAN_POINT ( 'NONE',  ( -24.64572710697934710, -6.998028550906933098, 47.88483805351501132 ) ) ;
#7044=VERTEX_POINT ( 'NONE', #8968 ) ;
#7051=ORIENTED_EDGE ( 'NONE', *, *, #14956, .T. ) ;
#7059=EDGE_CURVE ( 'NONE', #7490, #170, #14683, .T. ) ;
#7064=TOROIDAL_SURFACE ( 'NONE', #426, 9.500000000000001776, 0.5000000000000000000 ) ;
#7066=DIRECTION ( 'NONE',  ( -0.000000000000000000, -0.000000000000000000, 1.000000000000000000 ) ) ;
#7067=DIRECTION ( 'NONE',  ( 1.000000000000000000, 0.000000000000000000, 0.000000000000000000 ) ) ;
#7069=ORIENTED_EDGE ( 'NONE', *, *, #11053, .T. ) ;
#7071=ORIENTED_EDGE ( 'NONE', *, *, #5945, .F. ) ;
#7072=CARTESIAN_POINT ( 'NONE',  ( -3.190546569013415379, 0.8906624217387615339, -48.00000000000012079 ) ) ;
#7074=PLANE ( 'NONE',  #4705 ) ;
#7079=ORIENTED_EDGE ( 'NONE', *, *, #10546, .T. ) ;
#7086=CARTESIAN_POINT ( 'NONE',  ( -8.754378065084850391, 2.456381933588792865, 48.23869654929341522 ) ) ;
#7092=AXIS2_PLACEMENT_3D ( 'NONE', #2332, #12806, #5734 ) ;
#7099=CARTESIAN_POINT ( 'NONE',  ( -24.72817752516938228, 2.363221963240404566, -47.50000000000012079 ) ) ;
#7102=CARTESIAN_POINT ( 'NONE',  ( -8.537170960192302260, 2.067018546614597163, -48.00000000000012079 ) ) ;
#7113=DIRECTION ( 'NONE',  ( 0.000000000000000000, 0.000000000000000000, -1.000000000000000000 ) ) ;
#7114=ORIENTED_EDGE ( 'NONE', *, *, #214, .T. ) ;
#7125=CARTESIAN_POINT ( 'NONE',  ( -24.91597137788995298, -6.538835002183793321, 48.06338840812244939 ) ) ;
#7128=ORIENTED_EDGE ( 'NONE', *, *, #13338, .F. ) ;
#7132=AXIS2_PLACEMENT_3D ( 'NONE', #3716, #8424, #5811 ) ;
#7140=CARTESIAN_POINT ( 'NONE',  ( -16.99999999999998579, -2.249290599286303927, 50.00000000000012079 ) ) ;
#7141=DIRECTION ( 'NONE',  ( -0.8420378618367728718, -0.5394184268574404584, -0.000000000000000000 ) ) ;
#7147=VERTEX_POINT ( 'NONE', #13626 ) ;
#7148=DIRECTION ( 'NONE',  ( 0.5006040828730242698, -0.8656763553493063146, 0.000000000000000000 ) ) ;
#7149=ORIENTED_EDGE ( 'NONE', *, *, #6358, .F. ) ;
#7160=CARTESIAN_POINT ( 'NONE',  ( -9.394882438906904554, 2.563636819302931524, -48.00656353678737531 ) ) ;
#7165=ADVANCED_FACE ( 'NONE', ( #14706 ), #2000, .T. ) ;
#7166=TOROIDAL_SURFACE ( 'NONE', #2250, 3.694885682588112452, 0.5000000000000000000 ) ;
#7167=EDGE_LOOP ( 'NONE', ( #11484, #5134, #5295, #2696 ) ) ;
#7176=STYLED_ITEM('',(#15265),#14292);
#7178=CARTESIAN_POINT ( 'NONE',  ( -8.537170960192327129, 2.067018546614582508, 58.00000000000012079 ) ) ;
#7179=VECTOR ( 'NONE', #13305, 1000.000000000000000 ) ;
#7187=VERTEX_POINT ( 'NONE', #8856 ) ;
#7193=CIRCLE ( 'NONE', #545, 0.5000000000000000000 ) ;
#7195=CARTESIAN_POINT ( 'NONE',  ( -24.96222495693456978, -7.431276100536581275, -58.00000000000012079 ) ) ;
#7196=TOROIDAL_SURFACE ( 'NONE', #7441, 3.694885682588112452, 0.5000000000000000000 ) ;
#7197=DIRECTION ( 'NONE',  ( 0.000000000000000000, 0.000000000000000000, -1.000000000000000000 ) ) ;
#7201=AXIS2_PLACEMENT_3D ( 'NONE', #5999, #12924, #11756 ) ;
#7213=AXIS2_PLACEMENT_3D ( 'NONE', #3049, #6580, #3119 ) ;
#7217=CARTESIAN_POINT ( 'NONE',  ( -1.197457146693678753, -2.220571218158920335, 58.00000000000012079 ) ) ;
#7221=VERTEX_POINT ( 'NONE', #4465 ) ;
#7224=ORIENTED_EDGE ( 'NONE', *, *, #10388, .F. ) ;
#7235=DIRECTION ( 'NONE',  ( 1.224646799147353207E-16, -1.000000000000000000, 0.000000000000000000 ) ) ;
#7239=B_SPLINE_CURVE_WITH_KNOTS ( 'NONE', 3,
 ( #11768, #83, #10695, #1223, #5931, #10616, #6920, #3610, #8321, #151, #2540, #11915 ),
 .UNSPECIFIED., .F., .F.,
 ( 4, 2, 2, 2, 2, 4 ),
 ( 0.000000000000000000, 0.001071381053236910479, 0.002142762106473820958, 0.003214143159710731654, 0.003749833686329185484, 0.004285524212947640181 ),
 .UNSPECIFIED. ) ;
#7244=ORIENTED_EDGE ( 'NONE', *, *, #5245, .F. ) ;
#7246=EDGE_CURVE ( 'NONE', #4595, #8405, #4838, .T. ) ;
#7248=CARTESIAN_POINT ( 'NONE',  ( -1.197457146693715613, -2.220571218158943871, -48.50000000000012079 ) ) ;
#7256=CARTESIAN_POINT ( 'NONE',  ( -24.64146379341137560, -7.004861575982634037, 47.89606589046130125 ) ) ;
#7268=EDGE_CURVE ( 'NONE', #9532, #3566, #2416, .T. ) ;
#7270=CARTESIAN_POINT ( 'NONE',  ( -20.99999999999998579, -2.249290599286303483, 38.00000000000012079 ) ) ;
#7271=CIRCLE ( 'NONE', #5559, 0.4999999999999994449 ) ;
#7277=CARTESIAN_POINT ( 'NONE',  ( -16.99999999999998579, -2.249290599286303927, -57.50000000000012079 ) ) ;
#7283=DIRECTION ( 'NONE',  ( 0.8420378618367644341, 0.5394184268574535590, 0.000000000000000000 ) ) ;
#7292=ORIENTED_EDGE ( 'NONE', *, *, #11997, .T. ) ;
#7298=CYLINDRICAL_SURFACE ( 'NONE', #8606, 0.5000000000000001110 ) ;
#7303=CARTESIAN_POINT ( 'NONE',  ( -16.99999999999998579, -2.249290599286303927, 58.00000000000012079 ) ) ;
#7307=VERTEX_POINT ( 'NONE', #14248 ) ;
#7310=CARTESIAN_POINT ( 'NONE',  ( -21.58505662828840599, 4.908031226326156293, 57.50000000000012079 ) ) ;
#7311=EDGE_CURVE ( 'NONE', #9911, #7744, #12085, .T. ) ;
#7312=CARTESIAN_POINT ( 'NONE',  ( -3.190546569013415379, 0.8906624217387615339, 58.00000000000012079 ) ) ;
#7313=ORIENTED_EDGE ( 'NONE', *, *, #11839, .T. ) ;
#7315=CIRCLE ( 'NONE', #10258, 9.000000000000001776 ) ;
#7325=CARTESIAN_POINT ( 'NONE',  ( -8.982583014919022446, 1.839844381040865562, -47.50000000000012079 ) ) ;
#7339=ORIENTED_EDGE ( 'NONE', *, *, #4286, .T. ) ;
#7340=DIRECTION ( 'NONE',  ( 1.000000000000000000, 0.000000000000000000, 0.000000000000000000 ) ) ;
#7347=DIRECTION ( 'NONE',  ( -0.8586863916854874379, 0.5125013958363018318, 0.000000000000000000 ) ) ;
#7348=( BOUNDED_SURFACE ( )  B_SPLINE_SURFACE ( 3, 2, ( 
 ( #14561, #1634, #3023 ),
 ( #6334, #7713, #2715 ),
 ( #7557, #1568, #10955 ),
 ( #14626, #11026, #6480 ),
 ( #11169, #4078, #403 ),
 ( #1488, #478, #5104 ),
 ( #5255, #9811, #9952 ),
 ( #5402, #4468, #3607 ),
 ( #6625, #10095, #5718 ),
 ( #12635, #11463, #13713 ) ),
 .UNSPECIFIED., .F., .F., .F. ) 
 B_SPLINE_SURFACE_WITH_KNOTS ( ( 4, 2, 2, 2, 4 ),
 ( 3, 3 ),
 ( 0.0006711510808134562266, 0.001062132081067026709, 0.001453113081320596975, 0.001844094081574167241, 0.002235075081827737724 ),
 ( 0.000000000000000000, 1.000000000000000000 ),
 .UNSPECIFIED. ) 
 GEOMETRIC_REPRESENTATION_ITEM ( )  RATIONAL_B_SPLINE_SURFACE ( (
 ( 1.000000000000000000, 0.7254762501100212591, 1.000000000000000000),
 ( 1.000000000000000000, 0.7255094664176575670, 1.000000000000000000),
 ( 1.000000000000000000, 0.7239949553645330660, 1.000000000000000000),
 ( 1.000000000000000000, 0.7190573720639517052, 1.000000000000000000),
 ( 1.000000000000000000, 0.7156412189950384084, 1.000000000000000000),
 ( 1.000000000000000000, 0.7094102539595253942, 1.000000000000000000),
 ( 1.000000000000000000, 0.7066203625162220670, 1.000000000000000000),
 ( 1.000000000000000000, 0.7042417591948760824, 1.000000000000000000),
 ( 1.000000000000000000, 0.7046402682200600953, 1.000000000000000000),
 ( 1.000000000000000000, 0.7071067811865475727, 1.000000000000000000) ) ) 
 REPRESENTATION_ITEM ( '' )  SURFACE ( )  );
#7354=ADVANCED_FACE ( 'NONE', ( #319 ), #3034, .F. ) ;
#7356=ORIENTED_EDGE ( 'NONE', *, *, #4782, .F. ) ;
#7369=AXIS2_PLACEMENT_3D ( 'NONE', #12037, #8141, #12849 ) ;
#7378=DIRECTION ( 'NONE',  ( 0.000000000000000000, 0.000000000000000000, -1.000000000000000000 ) ) ;
#7382=CARTESIAN_POINT ( 'NONE',  ( -11.58528623411511305, -9.440246857018177451, 48.26816462195812818 ) ) ;
#7383=ORIENTED_EDGE ( 'NONE', *, *, #3030, .F. ) ;
#7385=VECTOR ( 'NONE', #8939, 1000.000000000000000 ) ;
#7398=VERTEX_POINT ( 'NONE', #8989 ) ;
#7404=CIRCLE ( 'NONE', #746, 0.5000000000000004441 ) ;
#7410=CIRCLE ( 'NONE', #282, 4.665819364273509073 ) ;
#7417=EDGE_CURVE ( 'NONE', #1375, #922, #13612, .T. ) ;
#7429=DIRECTION ( 'NONE',  ( 0.000000000000000000, 0.000000000000000000, 1.000000000000000000 ) ) ;
#7441=AXIS2_PLACEMENT_3D ( 'NONE', #7463, #14465, #3908 ) ;
#7449=DIRECTION ( 'NONE',  ( 0.000000000000000000, 0.000000000000000000, 1.000000000000000000 ) ) ;
#7454=ORIENTED_EDGE ( 'NONE', *, *, #10104, .T. ) ;
#7455=EDGE_LOOP ( 'NONE', ( #4107, #7128 ) ) ;
#7456=EDGE_CURVE ( 'NONE', #14789, #10204, #3400, .T. ) ;
#7457=CARTESIAN_POINT ( 'NONE',  ( -22.13891797369473480, 5.141277655368648780, 48.38337049880507834 ) ) ;
#7463=CARTESIAN_POINT ( 'NONE',  ( -30.80945343098651890, -5.389243620311580329, 57.50000000000012079 ) ) ;
#7469=DIRECTION ( 'NONE',  ( 1.000000000000000000, 0.000000000000000000, 0.000000000000000000 ) ) ;
#7473=CARTESIAN_POINT ( 'NONE',  ( -21.85476584171706449, 5.329050157244581420, 48.50000000000012079 ) ) ;
#7488=DIRECTION ( 'NONE',  ( 1.000000000000000000, 0.000000000000000000, 0.000000000000000000 ) ) ;
#7490=VERTEX_POINT ( 'NONE', #4138 ) ;
#7506=CARTESIAN_POINT ( 'NONE',  ( -9.090012166261184134, -7.380334305945262408, 48.00000000000014211 ) ) ;
#7520=DIRECTION ( 'NONE',  ( 0.000000000000000000, -0.000000000000000000, -1.000000000000000000 ) ) ;
#7527=ORIENTED_EDGE ( 'NONE', *, *, #12699, .F. ) ;
#7530=ADVANCED_FACE ( 'NONE', ( #673 ), #7817, .T. ) ;
#7533=DIRECTION ( 'NONE',  ( 0.8656763553492754504, 0.5006040828730772274, -1.896095000761754519E-14 ) ) ;
#7535=DIRECTION ( 'NONE',  ( 0.8420378618367727608, 0.5394184268574406804, 0.000000000000000000 ) ) ;
#7544=EDGE_CURVE ( 'NONE', #4976, #9584, #215, .T. ) ;
#7556=TOROIDAL_SURFACE ( 'NONE', #2879, 5.165819364273509073, 0.5000000000000000000 ) ;
#7557=CARTESIAN_POINT ( 'NONE',  ( -9.443282642412393457, 2.639297360524499592, 48.23807154671105479 ) ) ;
#7568=DIRECTION ( 'NONE',  ( 0.000000000000000000, 0.000000000000000000, -1.000000000000000000 ) ) ;
#7577=ORIENTED_EDGE ( 'NONE', *, *, #10069, .F. ) ;
#7579=ORIENTED_EDGE ( 'NONE', *, *, #5378, .F. ) ;
#7582=EDGE_CURVE ( 'NONE', #5046, #981, #5615, .T. ) ;
#7583=ADVANCED_FACE ( 'NONE', ( #12688 ), #3454, .T. ) ;
#7585=PRODUCT_DEFINITION ( 'UNKNOWN', '', #3869, #1353 ) ;
#7598=FACE_OUTER_BOUND ( 'NONE', #3831, .T. ) ;
#7599=DIRECTION ( 'NONE',  ( -0.000000000000000000, -0.000000000000000000, -1.000000000000000000 ) ) ;
#7602=CARTESIAN_POINT ( 'NONE',  ( -25.99999999999998934, -2.249290599286303927, 47.50000000000012079 ) ) ;
#7611=DIRECTION ( 'NONE',  ( 0.000000000000000000, -0.000000000000000000, -1.000000000000000000 ) ) ;
#7613=VERTEX_POINT ( 'NONE', #3375 ) ;
#7617=ORIENTED_EDGE ( 'NONE', *, *, #5696, .F. ) ;
#7620=TOROIDAL_SURFACE ( 'NONE', #486, 3.694885682587998765, 0.5000000000000000000 ) ;
#7624=VERTEX_POINT ( 'NONE', #15149 ) ;
#7630=TOROIDAL_SURFACE ( 'NONE', #11551, 3.694885682587998765, 0.5000000000000000000 ) ;
#7632=EDGE_CURVE ( 'NONE', #864, #10987, #1437, .T. ) ;
#7634=DIRECTION ( 'NONE',  ( 0.8656763553493062036, 0.5006040828730242698, 0.000000000000000000 ) ) ;
#7642=ORIENTED_EDGE ( 'NONE', *, *, #7059, .F. ) ;
#7645=AXIS2_PLACEMENT_3D ( 'NONE', #11369, #10384, #9071 ) ;
#7646=FACE_OUTER_BOUND ( 'NONE', #12487, .T. ) ;
#7648=CARTESIAN_POINT ( 'NONE',  ( -25.22031829551916360, -6.987901215495521789, -48.36903577193041315 ) ) ;
#7653=EDGE_CURVE ( 'NONE', #3003, #2288, #10538, .T. ) ;
#7657=VERTEX_POINT ( 'NONE', #7993 ) ;
#7659=CARTESIAN_POINT ( 'NONE',  ( -8.842479278987921631, -7.118053859731281463, 48.00000000000012079 ) ) ;
#7660=CARTESIAN_POINT ( 'NONE',  ( -12.41494337171168283, -9.406612424898836977, 57.50000000000012079 ) ) ;
#7667=CARTESIAN_POINT ( 'NONE',  ( -21.66581936427349575, -2.249290599286303483, 57.50000000000012079 ) ) ;
#7671=EDGE_CURVE ( 'NONE', #7044, #8826, #2633, .T. ) ;
#7673=ORIENTED_EDGE ( 'NONE', *, *, #10360, .F. ) ;
#7679=DIRECTION ( 'NONE',  ( 0.8586863916854811096, -0.5125013958363124900, 0.000000000000000000 ) ) ;
#7686=AXIS2_PLACEMENT_3D ( 'NONE', #5318, #10016, #13546 ) ;
#7696=ORIENTED_EDGE ( 'NONE', *, *, #4673, .F. ) ;
#7704=CARTESIAN_POINT ( 'NONE',  ( -8.537170960192302260, 2.067018546614596719, -48.00000000000012079 ) ) ;
#7713=CARTESIAN_POINT ( 'NONE',  ( -9.198099345814858552, 2.262399347264687943, 48.43121057161710041 ) ) ;
#7716=DIRECTION ( 'NONE',  ( -0.000000000000000000, -0.000000000000000000, 1.000000000000000000 ) ) ;
#7723=EDGE_CURVE ( 'NONE', #3752, #4049, #10738, .T. ) ;
#7729=DIRECTION ( 'NONE',  ( -1.000000000000000000, 0.000000000000000000, 0.000000000000000000 ) ) ;
#7744=VERTEX_POINT ( 'NONE', #4767 ) ;
#7750=DIRECTION ( 'NONE',  ( -0.8420378618367644341, -0.5394184268574535590, 0.000000000000000000 ) ) ;
#7752=EDGE_CURVE ( 'NONE', #9584, #3003, #11722, .T. ) ;
#7756=DIRECTION ( 'NONE',  ( -1.000000000000000000, 0.000000000000000000, 0.000000000000000000 ) ) ;
#7757=VERTEX_POINT ( 'NONE', #8311 ) ;
#7759=EDGE_CURVE ( 'NONE', #3759, #14513, #6005, .T. ) ;
#7760=DIRECTION ( 'NONE',  ( 0.5006040828730242698, -0.8656763553493062036, 0.000000000000000000 ) ) ;
#7761=CARTESIAN_POINT ( 'NONE',  ( -25.04138923958014473, -6.321889167469157300, -58.00000000000012079 ) ) ;
#7771=DIRECTION ( 'NONE',  ( -0.5394184268574520047, 0.8420378618367654333, 0.000000000000000000 ) ) ;
#7772=CARTESIAN_POINT ( 'NONE',  ( -8.537170960192302260, 2.067018546614596719, 48.00000000000012079 ) ) ;
#7780=DIRECTION ( 'NONE',  ( 0.000000000000000000, 0.000000000000000000, 1.000000000000000000 ) ) ;
#7781=CARTESIAN_POINT ( 'NONE',  ( -9.456839514482961562, 2.659958822950721835, 48.50000000000012079 ) ) ;
#7785=CIRCLE ( 'NONE', #3111, 3.694885682587998765 ) ;
#7786=VECTOR ( 'NONE', #1588, 1000.000000000000000 ) ;
#7791=DIRECTION ( 'NONE',  ( -0.8656763553493062036, -0.5006040828730242698, -0.000000000000000000 ) ) ;
#7800=CARTESIAN_POINT ( 'NONE',  ( -24.83354747574476207, -6.700581361908810152, -48.23896987259369240 ) ) ;
#7809=VECTOR ( 'NONE', #7791, 1000.000000000000000 ) ;
#7810=EDGE_LOOP ( 'NONE', ( #11396, #7339, #11607, #825 ) ) ;
#7811=DIRECTION ( 'NONE',  ( -0.8656763553493062036, -0.5006040828730242698, -0.000000000000000000 ) ) ;
#7817=TOROIDAL_SURFACE ( 'NONE', #3143, 8.500000000000000000, 0.5000000000000000000 ) ;
#7820=CARTESIAN_POINT ( 'NONE',  ( -3.190546569013415379, 0.8906624217387615339, 57.50000000000012079 ) ) ;
#7825=EDGE_LOOP ( 'NONE', ( #3974, #509, #2100, #5314 ) ) ;
#7828=EDGE_LOOP ( 'NONE', ( #3994, #10288, #1761, #12700 ) ) ;
#7830=ORIENTED_EDGE ( 'NONE', *, *, #165, .T. ) ;
#7836=ORIENTED_EDGE ( 'NONE', *, *, #2638, .T. ) ;
#7840=CARTESIAN_POINT ( 'NONE',  ( -10.08688311991301312, -8.022742138608869311, 47.66502101098957667 ) ) ;
#7852=CARTESIAN_POINT ( 'NONE',  ( -22.46208338003149407, 4.939996070762163960, -48.38299871081639481 ) ) ;
#7865=CIRCLE ( 'NONE', #5663, 3.694885682587998765 ) ;
#7866=DIRECTION ( 'NONE',  ( 1.000000000000000000, 0.000000000000000000, 0.000000000000000000 ) ) ;
#7870=CARTESIAN_POINT ( 'NONE',  ( -3.285520523749251520, 5.681530634151883419, -48.50000000000012079 ) ) ;
#7874=DIRECTION ( 'NONE',  ( 1.000000000000000000, 0.000000000000000000, -0.000000000000000000 ) ) ;
#7875=DIRECTION ( 'NONE',  ( -0.000000000000000000, -0.000000000000000000, 1.000000000000000000 ) ) ;
#7878=ORIENTED_EDGE ( 'NONE', *, *, #1031, .T. ) ;
#7880=EDGE_CURVE ( 'NONE', #13865, #4611, #1877, .T. ) ;
#7882=VERTEX_POINT ( 'NONE', #8735 ) ;
#7889=AXIS2_PLACEMENT_3D ( 'NONE', #3578, #6128, #7347 ) ;
#7891=DIRECTION ( 'NONE',  ( 0.000000000000000000, -0.000000000000000000, -1.000000000000000000 ) ) ;
#7902=ORIENTED_EDGE ( 'NONE', *, *, #6998, .F. ) ;
#7916=VECTOR ( 'NONE', #3725, 1000.000000000000114 ) ;
#7919=DIRECTION ( 'NONE',  ( -1.000000000000000000, 0.000000000000000000, 0.000000000000000000 ) ) ;
#7921=EDGE_CURVE ( 'NONE', #2105, #7961, #10499, .T. ) ;
#7923=DIRECTION ( 'NONE',  ( -0.5006040828730989878, 0.8656763553492631269, 0.000000000000000000 ) ) ;
#7924=ORIENTED_EDGE ( 'NONE', *, *, #6045, .F. ) ;
#7925=DIRECTION ( 'NONE',  ( 0.5125013958363011657, 0.8586863916854879930, -0.000000000000000000 ) ) ;
#7926=ORIENTED_EDGE ( 'NONE', *, *, #7632, .F. ) ;
#7932=DIRECTION ( 'NONE',  ( -0.000000000000000000, 0.000000000000000000, 1.000000000000000000 ) ) ;
#7935=DIRECTION ( 'NONE',  ( -1.000000000000000000, 0.000000000000000000, 0.000000000000000000 ) ) ;
#7949=DIRECTION ( 'NONE',  ( -0.5454721580263366398, 0.8381289428352246551, 4.385647630081457888E-16 ) ) ;
#7961=VERTEX_POINT ( 'NONE', #6736 ) ;
#7965=AXIS2_PLACEMENT_3D ( 'NONE', #10063, #14747, #3288 ) ;
#7976=CARTESIAN_POINT ( 'NONE',  ( -16.99999999999998579, -2.249290599286303927, -48.00000000000012079 ) ) ;
#7993=CARTESIAN_POINT ( 'NONE',  ( -28.95977857253358323, -8.587818791446787614, 48.00000000000012079 ) ) ;
#7994=VERTEX_POINT ( 'NONE', #14366 ) ;
#7996=ORIENTED_EDGE ( 'NONE', *, *, #7653, .F. ) ;
#8010=ORIENTED_EDGE ( 'NONE', *, *, #6370, .F. ) ;
#8011=DIRECTION ( 'NONE',  ( 0.4543483311474731945, -0.8908241094534353754, -0.000000000000000000 ) ) ;
#8020=CARTESIAN_POINT ( 'NONE',  ( -9.426221351844976226, -7.120495567270975101, -47.92899112040988996 ) ) ;
#8022=ORIENTED_EDGE ( 'NONE', *, *, #10410, .F. ) ;
#8030=CIRCLE ( 'NONE', #14428, 0.5000000000000001110 ) ;
#8034=AXIS2_PLACEMENT_3D ( 'NONE', #14592, #5435, #6583 ) ;
#8039=CARTESIAN_POINT ( 'NONE',  ( -1.197457146693684082, -2.220571218158921223, 58.00000000000012079 ) ) ;
#8042=AXIS2_PLACEMENT_3D ( 'NONE', #9433, #13191, #4959 ) ;
#8059=EDGE_CURVE ( 'NONE', #5398, #10712, #5331, .T. ) ;
#8070=AXIS2_PLACEMENT_3D ( 'NONE', #2160, #8011, #8252 ) ;
#8071=ORIENTED_EDGE ( 'NONE', *, *, #12312, .F. ) ;
#8072=DIRECTION ( 'NONE',  ( -0.000000000000000000, -0.000000000000000000, 1.000000000000000000 ) ) ;
#8075=TOROIDAL_SURFACE ( 'NONE', #2171, 9.500000000000001776, 0.5000000000000000000 ) ;
#8076=ORIENTED_EDGE ( 'NONE', *, *, #1823, .T. ) ;
#8082=DIRECTION ( 'NONE',  ( 0.4543483311474630915, -0.8908241094534405935, 0.000000000000000000 ) ) ;
#8094=AXIS2_PLACEMENT_3D ( 'NONE', #4088, #7568, #13487 ) ;
#8096=AXIS2_PLACEMENT_3D ( 'NONE', #2094, #2413, #6954 ) ;
#8099=CARTESIAN_POINT ( 'NONE',  ( -9.855956283963589470, -8.104443761338727015, -48.08251050686958905 ) ) ;
#8106=DIRECTION ( 'NONE',  ( 1.000000000000000000, 0.000000000000000000, 0.000000000000000000 ) ) ;
#8108=DIRECTION ( 'NONE',  ( -0.000000000000000000, 0.000000000000000000, 1.000000000000000000 ) ) ;
#8112=VERTEX_POINT ( 'NONE', #9599 ) ;
#8114=ORIENTED_EDGE ( 'NONE', *, *, #13641, .T. ) ;
#8119=CARTESIAN_POINT ( 'NONE',  ( -7.999999999999986677, -2.249290599286305259, -47.50000000000012079 ) ) ;
#8122=CARTESIAN_POINT ( 'NONE',  ( -5.040221427466046400, 4.089237592873870675, 48.00000000000012079 ) ) ;
#8127=CARTESIAN_POINT ( 'NONE',  ( -24.12883632398703782, 3.619414784477793301, -48.08465436988272756 ) ) ;
#8132=CARTESIAN_POINT ( 'NONE',  ( -16.99999999999998579, -2.249290599286303927, 50.50000000000012079 ) ) ;
#8140=ORIENTED_EDGE ( 'NONE', *, *, #1031, .F. ) ;
#8141=DIRECTION ( 'NONE',  ( 0.000000000000000000, 0.000000000000000000, -1.000000000000000000 ) ) ;
#8147=CARTESIAN_POINT ( 'NONE',  ( -12.14523415828302078, -9.827631355817260328, 48.50000000000012079 ) ) ;
#8152=DIRECTION ( 'NONE',  ( 1.000000000000000000, 0.000000000000000000, 0.000000000000000000 ) ) ;
#8153=ORIENTED_EDGE ( 'NONE', *, *, #7723, .T. ) ;
#8157=TOROIDAL_SURFACE ( 'NONE', #1521, 4.165819364273509962, 0.5000000000000000000 ) ;
#8161=AXIS2_PLACEMENT_3D ( 'NONE', #2834, #9927, #455 ) ;
#8167=DIRECTION ( 'NONE',  ( 1.224646799147353207E-16, 1.000000000000000000, 0.000000000000000000 ) ) ;
#8176=AXIS2_PLACEMENT_3D ( 'NONE', #13634, #776, #3403 ) ;
#8179=DIRECTION ( 'NONE',  ( -0.000000000000000000, 0.000000000000000000, 1.000000000000000000 ) ) ;
#8192=DIRECTION ( 'NONE',  ( 0.8656763553493062036, 0.5006040828730242698, 0.000000000000000000 ) ) ;
#8199=ADVANCED_FACE ( 'NONE', ( #11111 ), #2809, .T. ) ;
#8202=EDGE_CURVE ( 'NONE', #1125, #8531, #4173, .T. ) ;
#8204=ORIENTED_EDGE ( 'NONE', *, *, #12039, .F. ) ;
#8206=CARTESIAN_POINT ( 'NONE',  ( -9.037775043065352065, 2.932694901963889489, 58.00000000000012079 ) ) ;
#8222=VERTEX_POINT ( 'NONE', #12650 ) ;
#8232=FACE_OUTER_BOUND ( 'NONE', #13725, .T. ) ;
#8244=DIRECTION ( 'NONE',  ( 0.000000000000000000, 0.000000000000000000, -1.000000000000000000 ) ) ;
#8247=DIRECTION ( 'NONE',  ( 0.000000000000000000, 0.000000000000000000, 1.000000000000000000 ) ) ;
#8248=DIRECTION ( 'NONE',  ( 0.8420378618367651002, 0.5394184268574528929, -2.807225425332302624E-15 ) ) ;
#8249=FACE_OUTER_BOUND ( 'NONE', #5652, .T. ) ;
#8252=DIRECTION ( 'NONE',  ( -0.8908241094534361526, -0.4543483311474716957, 0.000000000000000000 ) ) ;
#8257=EDGE_CURVE ( 'NONE', #3688, #2288, #11050, .T. ) ;
#8258=ADVANCED_FACE ( 'NONE', ( #5502 ), #10112, .T. ) ;
#8265=DIRECTION ( 'NONE',  ( 0.5394184268574402363, -0.8420378618367729828, 0.000000000000000000 ) ) ;
#8269=CARTESIAN_POINT ( 'NONE',  ( -24.60511756109301373, -7.062218017875619758, -48.00656353678737531 ) ) ;
#8274=ORIENTED_EDGE ( 'NONE', *, *, #8518, .T. ) ;
#8277=DIRECTION ( 'NONE',  ( -0.8656763553492640151, -0.5006040828730974335, 0.000000000000000000 ) ) ;
#8284=CARTESIAN_POINT ( 'NONE',  ( -24.85140262670387301, -6.666068128078234345, 48.18452149279842445 ) ) ;
#8287=ADVANCED_FACE ( 'NONE', ( #3180 ), #789, .T. ) ;
#8303=CIRCLE ( 'NONE', #10015, 0.5000000000000004441 ) ;
#8304=EDGE_CURVE ( 'NONE', #56, #4994, #7865, .T. ) ;
#8306=CIRCLE ( 'NONE', #10999, 4.665819364273509073 ) ;
#8307=FACE_OUTER_BOUND ( 'NONE', #8598, .T. ) ;
#8311=CARTESIAN_POINT ( 'NONE',  ( -1.197457146693678531, -2.220571218158920779, -48.00000000000012079 ) ) ;
#8314=VECTOR ( 'NONE', #219, 1000.000000000000000 ) ;
#8319=CIRCLE ( 'NONE', #10530, 3.694885682587998765 ) ;
#8321=CARTESIAN_POINT ( 'NONE',  ( -22.41471376588497222, 4.941665658445489662, -48.26816462195809265 ) ) ;
#8327=EDGE_LOOP ( 'NONE', ( #7383, #6941 ) ) ;
#8328=DIRECTION ( 'NONE',  ( -1.000000000000000000, 0.000000000000000000, 0.000000000000000000 ) ) ;
#8337=ORIENTED_EDGE ( 'NONE', *, *, #7246, .T. ) ;
#8339=DIRECTION ( 'NONE',  ( 0.5394184268574520047, -0.8420378618367654333, 0.000000000000000000 ) ) ;
#8344=CARTESIAN_POINT ( 'NONE',  ( 0.5043391135745837195, 0.8906624217387615339, -57.50000000000012079 ) ) ;
#8362=CARTESIAN_POINT ( 'NONE',  ( -24.99086469133269617, -6.390485686409522081, 48.00342231809331395 ) ) ;
#8373=CARTESIAN_POINT ( 'NONE',  ( -3.285520523749251520, 5.681530634151883419, 48.50000000000012079 ) ) ;
#8376=CARTESIAN_POINT ( 'NONE',  ( -24.90998783373886738, 2.881753107372537759, 48.00000000000012079 ) ) ;
#8382=ORIENTED_EDGE ( 'NONE', *, *, #1309, .T. ) ;
#8385=DIRECTION ( 'NONE',  ( -0.8656763553493062036, -0.5006040828730242698, -0.000000000000000000 ) ) ;
#8395=CARTESIAN_POINT ( 'NONE',  ( -8.590985667557523797, 2.187759657648595368, 48.00000000000012079 ) ) ;
#8396=VERTEX_POINT ( 'NONE', #4728 ) ;
#8400=CARTESIAN_POINT ( 'NONE',  ( -9.268887740808379405, 2.359106894006888666, -47.70917337021941762 ) ) ;
#8401=CARTESIAN_POINT ( 'NONE',  ( -7.499999999999985789, -2.249290599286303927, -48.00000000000012079 ) ) ;
#8403=CARTESIAN_POINT ( 'NONE',  ( -22.46208338003149407, 4.939996070762163960, 48.38299871081639481 ) ) ;
#8404=VECTOR ( 'NONE', #5418, 1000.000000000000114 ) ;
#8405=VERTEX_POINT ( 'NONE', #11797 ) ;
#8409=ORIENTED_EDGE ( 'NONE', *, *, #6585, .F. ) ;
#8421=CARTESIAN_POINT ( 'NONE',  ( -24.89835624542414649, -6.565460432723037698, 47.52815511422343775 ) ) ;
#8424=DIRECTION ( 'NONE',  ( -0.000000000000000000, 0.000000000000000000, 1.000000000000000000 ) ) ;
#8436=LINE ( 'NONE', #13126, #9394 ) ;
#8438=ADVANCED_FACE ( 'NONE', ( #1337 ), #11284, .F. ) ;
#8450=ORIENTED_EDGE ( 'NONE', *, *, #11499, .T. ) ;
#8456=ADVANCED_FACE ( 'NONE', ( #13186 ), #7620, .T. ) ;
#8458=CIRCLE ( 'NONE', #9921, 0.5000000000000008882 ) ;
#8461=CARTESIAN_POINT ( 'NONE',  ( -23.85820543185402798, 3.853856159079054322, 48.12676452506695313 ) ) ;
#8472=CARTESIAN_POINT ( 'NONE',  ( -10.31873516982594907, -8.289185193041582522, 47.74939190649462972 ) ) ;
#8475=DIRECTION ( 'NONE',  ( -0.8381289428352193260, -0.5454721580263449665, 0.000000000000000000 ) ) ;
#8476=ADVANCED_FACE ( 'NONE', ( #8778 ), #9093, .T. ) ;
#8477=ORIENTED_EDGE ( 'NONE', *, *, #1492, .F. ) ;
#8480=FACE_OUTER_BOUND ( 'NONE', #9850, .T. ) ;
#8482=CARTESIAN_POINT ( 'NONE',  ( -21.85476584171706449, 5.329050157244580532, 48.50000000000012079 ) ) ;
#8486=LINE ( 'NONE', #12521, #1133 ) ;
#8492=CARTESIAN_POINT ( 'NONE',  ( -8.779681704480811533, 2.489320016922789147, -48.36903577193039894 ) ) ;
#8503=DIRECTION ( 'NONE',  ( 0.5006040828730228265, -0.8656763553493070917, 0.000000000000000000 ) ) ;
#8507=CARTESIAN_POINT ( 'NONE',  ( -24.80190064845255193, -6.760980556683136911, 48.50000000000010658 ) ) ;
#8516=CARTESIAN_POINT ( 'NONE',  ( -10.14179456814604130, -8.352437357651758987, 48.12676452506694602 ) ) ;
#8518=EDGE_CURVE ( 'NONE', #13079, #3246, #250, .T. ) ;
#8526=EDGE_LOOP ( 'NONE', ( #6278, #10537, #2437, #616 ) ) ;
#8531=VERTEX_POINT ( 'NONE', #5031 ) ;
#8532=CARTESIAN_POINT ( 'NONE',  ( -21.85476584171713199, 5.329050157244537900, 48.50000000000012079 ) ) ;
#8537=CARTESIAN_POINT ( 'NONE',  ( -28.95977857253364007, -8.587818791446682809, 58.00000000000012079 ) ) ;
#8542=CARTESIAN_POINT ( 'NONE',  ( -16.99999999999998579, -2.249290599286303927, -47.50000000000012079 ) ) ;
#8545=DIRECTION ( 'NONE',  ( 1.000000000000000000, 0.000000000000000000, 0.000000000000000000 ) ) ;
#8548=ADVANCED_FACE ( 'NONE', ( #13263 ), #7348, .F. ) ;
#8549=ORIENTED_EDGE ( 'NONE', *, *, #3417, .T. ) ;
#8555=CARTESIAN_POINT ( 'NONE',  ( -0.9277479332649583021, -2.641590149077306826, 48.50000000000012079 ) ) ;
#8556=CARTESIAN_POINT ( 'NONE',  ( -8.593267841128518825, 2.185894787177926624, -48.01308457333531265 ) ) ;
#8567=DIRECTION ( 'NONE',  ( 0.000000000000000000, 0.000000000000000000, 1.000000000000000000 ) ) ;
#8576=FACE_OUTER_BOUND ( 'NONE', #11650, .T. ) ;
#8585=DIRECTION ( 'NONE',  ( -0.000000000000000000, -0.000000000000000000, 1.000000000000000000 ) ) ;
#8590=ADVANCED_FACE ( 'NONE', ( #5635 ), #4167, .T. ) ;
#8593=AXIS2_PLACEMENT_3D ( 'NONE', #11597, #3212, #6905 ) ;
#8598=EDGE_LOOP ( 'NONE', ( #6615, #373, #7079, #4566 ) ) ;
#8606=AXIS2_PLACEMENT_3D ( 'NONE', #11987, #8385, #7148 ) ;
#8609=EDGE_CURVE ( 'NONE', #11451, #10712, #9178, .T. ) ;
#8610=EDGE_CURVE ( 'NONE', #10346, #1708, #10246, .T. ) ;
#8615=CARTESIAN_POINT ( 'NONE',  ( -23.68178719075091365, 3.790042057515504048, 47.74919337097016836 ) ) ;
#8616=ORIENTED_EDGE ( 'NONE', *, *, #7456, .F. ) ;
#8628=CARTESIAN_POINT ( 'NONE',  ( -8.787473001628837821, 2.499856724289235554, -48.50000000000012079 ) ) ;
#8630=DIRECTION ( 'NONE',  ( 1.000000000000000000, -3.565820478396769525E-15, 0.000000000000000000 ) ) ;
#8634=ORIENTED_EDGE ( 'NONE', *, *, #14956, .F. ) ;
#8648=ADVANCED_FACE ( 'NONE', ( #13862 ), #13781, .T. ) ;
#8660=ADVANCED_FACE ( 'NONE', ( #303 ), #7298, .T. ) ;
#8662=ORIENTED_EDGE ( 'NONE', *, *, #3917, .F. ) ;
#8667=VECTOR ( 'NONE', #11593, 1000.000000000000000 ) ;
#8669=EDGE_LOOP ( 'NONE', ( #7051, #10385, #4899, #4531 ) ) ;
#8681=AXIS2_PLACEMENT_3D ( 'NONE', #10705, #162, #9561 ) ;
#8682=CARTESIAN_POINT ( 'NONE',  ( -9.037775043065352065, 2.932694901963889489, -57.50000000000012079 ) ) ;
#8683=ORIENTED_EDGE ( 'NONE', *, *, #5426, .T. ) ;
#8686=FACE_OUTER_BOUND ( 'NONE', #2024, .T. ) ;
#8693=ADVANCED_FACE ( 'NONE', ( #1295 ), #7630, .T. ) ;
#8705=DIRECTION ( 'NONE',  ( -0.000000000000000000, 0.000000000000000000, 1.000000000000000000 ) ) ;
#8711=DIRECTION ( 'NONE',  ( -0.000000000000000000, 0.000000000000000000, 1.000000000000000000 ) ) ;
#8717=ORIENTED_EDGE ( 'NONE', *, *, #1309, .F. ) ;
#8720=LINE ( 'NONE', #14645, #4719 ) ;
#8734=ORIENTED_EDGE ( 'NONE', *, *, #11279, .F. ) ;
#8735=CARTESIAN_POINT ( 'NONE',  ( -12.33418063572647938, -2.249290599286303927, -57.50000000000012079 ) ) ;
#8743=CARTESIAN_POINT ( 'NONE',  ( -9.037775043065352065, 2.932694901963889489, 57.50000000000012079 ) ) ;
#8756=EDGE_LOOP ( 'NONE', ( #443, #9563, #5337, #2163 ) ) ;
#8763=AXIS2_PLACEMENT_3D ( 'NONE', #3658, #14274, #7340 ) ;
#8773=CYLINDRICAL_SURFACE ( 'NONE', #7686, 9.000000000000001776 ) ;
#8776=AXIS2_PLACEMENT_3D ( 'NONE', #4145, #1767, #5239 ) ;
#8778=FACE_OUTER_BOUND ( 'NONE', #8756, .T. ) ;
#8783=DIRECTION ( 'NONE',  ( -0.5006040828730242698, 0.8656763553493063146, 0.000000000000000000 ) ) ;
#8787=CIRCLE ( 'NONE', #9298, 3.694885682587998765 ) ;
#8789=CARTESIAN_POINT ( 'NONE',  ( -3.190546569013415379, 0.8906624217387615339, 57.50000000000012079 ) ) ;
#8793=CARTESIAN_POINT ( 'NONE',  ( -32.80254285330622110, -2.278009980413880697, -48.00000000000012079 ) ) ;
#8794=LINE ( 'NONE', #13491, #1754 ) ;
#8799=DIRECTION ( 'NONE',  ( -0.8420378618367675427, -0.5394184268574490071, -0.000000000000000000 ) ) ;
#8800=CARTESIAN_POINT ( 'NONE',  ( -16.99999999999998579, -2.249290599286303927, 38.50000000000012790 ) ) ;
#8815=ORIENTED_EDGE ( 'NONE', *, *, #4559, .T. ) ;
#8816=AXIS2_PLACEMENT_3D ( 'NONE', #3175, #7875, #12567 ) ;
#8824=EDGE_LOOP ( 'NONE', ( #13773, #7454, #34, #3418 ) ) ;
#8826=VERTEX_POINT ( 'NONE', #5365 ) ;
#8829=DIRECTION ( 'NONE',  ( -1.000000000000000000, 0.000000000000000000, 0.000000000000000000 ) ) ;
#8835=ADVANCED_FACE ( 'NONE', ( #7598 ), #12211, .T. ) ;
#8847=CARTESIAN_POINT ( 'NONE',  ( -11.58528623411511305, -9.440246857018177451, -48.26816462195812818 ) ) ;
#8849=VERTEX_POINT ( 'NONE', #12519 ) ;
#8853=CIRCLE ( 'NONE', #6164, 5.165819364273509073 ) ;
#8856=CARTESIAN_POINT ( 'NONE',  ( -7.999999999999986677, -2.249290599286302594, 38.50000000000012790 ) ) ;
#8857=EDGE_CURVE ( 'NONE', #15020, #7147, #1485, .T. ) ;
#8863=CARTESIAN_POINT ( 'NONE',  ( -16.99999999999998579, -2.249290599286303927, 38.50000000000012790 ) ) ;
#8865=LINE ( 'NONE', #13561, #13905 ) ;
#8867=CARTESIAN_POINT ( 'NONE',  ( -16.99999999999998579, -2.249290599286303927, -57.50000000000012079 ) ) ;
#8874=CARTESIAN_POINT ( 'NONE',  ( -21.85476584171713199, 5.329050157244537900, 48.00000000000012079 ) ) ;
#8880=CARTESIAN_POINT ( 'NONE',  ( -3.190546569013415379, 0.8906624217387615339, -48.00000000000012079 ) ) ;
#8884=EDGE_CURVE ( 'NONE', #2664, #14041, #8853, .T. ) ;
#8885=VECTOR ( 'NONE', #14925, 1000.000000000000000 ) ;
#8891=VECTOR ( 'NONE', #9826, 1000.000000000000000 ) ;
#8898=DIRECTION ( 'NONE',  ( 0.5394184268574520047, -0.8420378618367654333, 0.000000000000000000 ) ) ;
#8899=EDGE_CURVE ( 'NONE', #10987, #11056, #14508, .T. ) ;
#8900=EDGE_CURVE ( 'NONE', #981, #7221, #3359, .T. ) ;
#8911=CARTESIAN_POINT ( 'NONE',  ( -25.21252699837112132, -6.998437922861947769, 57.50000000000012079 ) ) ;
#8914=SHAPE_REPRESENTATION ( 'Plastic-Headed Retaining Pin', ( #6315 ), #9517 ) ;
#8918=VERTEX_POINT ( 'NONE', #5599 ) ;
#8919=CIRCLE ( 'NONE', #7201, 0.4999999999999995559 ) ;
#8920=ORIENTED_EDGE ( 'NONE', *, *, #8202, .F. ) ;
#8921=CIRCLE ( 'NONE', #8681, 4.165819364273509962 ) ;
#8924=CARTESIAN_POINT ( 'NONE',  ( -24.34296084301338681, 2.966536634491813818, -47.54128347412125066 ) ) ;
#8928=DIRECTION ( 'NONE',  ( 1.000000000000000000, 0.000000000000000000, 0.000000000000000000 ) ) ;
#8929=CIRCLE ( 'NONE', #4251, 1.000000000000000888 ) ;
#8932=CARTESIAN_POINT ( 'NONE',  ( -9.101643754575787781, 2.066879234150345024, 47.52815511422343775 ) ) ;
#8939=DIRECTION ( 'NONE',  ( -0.8420378618367644341, -0.5394184268574535590, -0.000000000000000000 ) ) ;
#8948=EDGE_CURVE ( 'NONE', #981, #13646, #12805, .T. ) ;
#8964=DIRECTION ( 'NONE',  ( 0.000000000000000000, 0.000000000000000000, -1.000000000000000000 ) ) ;
#8967=EDGE_CURVE ( 'NONE', #5398, #6058, #12568, .T. ) ;
#8968=CARTESIAN_POINT ( 'NONE',  ( -24.12409601409935078, -6.885803942510236197, -58.00000000000012079 ) ) ;
#8972=CARTESIAN_POINT ( 'NONE',  ( -16.99999999999998579, -2.249290599286303927, -50.50000000000012079 ) ) ;
#8973=ORIENTED_EDGE ( 'NONE', *, *, #349, .T. ) ;
#8976=DIRECTION ( 'NONE',  ( -0.8656763553493069807, -0.5006040828730229375, -0.000000000000000000 ) ) ;
#8979=CARTESIAN_POINT ( 'NONE',  ( -5.040221427466112125, 4.089237592873837812, -57.50000000000012079 ) ) ;
#8984=ADVANCED_FACE ( 'NONE', ( #12341 ), #2021, .F. ) ;
#8987=ORIENTED_EDGE ( 'NONE', *, *, #6868, .F. ) ;
#8989=CARTESIAN_POINT ( 'NONE',  ( -9.875903985900574611, 2.387222743937553293, -58.00000000000012079 ) ) ;
#8990=VERTEX_POINT ( 'NONE', #4248 ) ;
#8996=CARTESIAN_POINT ( 'NONE',  ( -23.03920594196030791, 4.522656845271360915, -48.26696389624889605 ) ) ;
#9004=DIRECTION ( 'NONE',  ( 0.000000000000000000, 0.000000000000000000, -1.000000000000000000 ) ) ;
#9009=CIRCLE ( 'NONE', #169, 4.665819364273509073 ) ;
#9017=VERTEX_POINT ( 'NONE', #8793 ) ;
#9023=CIRCLE ( 'NONE', #8763, 9.500000000000001776 ) ;
#9024=CARTESIAN_POINT ( 'NONE',  ( -8.509932750408504276, 13.28409490805591808, -57.50000000000012079 ) ) ;
#9030=ORIENTED_EDGE ( 'NONE', *, *, #10425, .T. ) ;
#9034=DIRECTION ( 'NONE',  ( -0.000000000000000000, -0.000000000000000000, 1.000000000000000000 ) ) ;
#9036=CIRCLE ( 'NONE', #13458, 0.5000000000000004441 ) ;
#9049=AXIS2_PLACEMENT_3D ( 'NONE', #2092, #10421, #7023 ) ;
#9055=CARTESIAN_POINT ( 'NONE',  ( -16.99999999999998579, -2.249290599286303927, -57.50000000000012079 ) ) ;
#9057=DIRECTION ( 'NONE',  ( 1.000000000000000000, 0.000000000000000000, 0.000000000000000000 ) ) ;
#9059=DIRECTION ( 'NONE',  ( -0.000000000000000000, -0.000000000000000000, 1.000000000000000000 ) ) ;
#9060=CARTESIAN_POINT ( 'NONE',  ( 1.004339113574583608, 0.8906624217387615339, -48.50000000000012079 ) ) ;
#9061=CARTESIAN_POINT ( 'NONE',  ( -30.80945343098651890, -5.389243620311580329, -48.00000000000012079 ) ) ;
#9062=ORIENTED_EDGE ( 'NONE', *, *, #8, .F. ) ;
#9063=DIRECTION ( 'NONE',  ( 0.000000000000000000, 0.000000000000000000, -1.000000000000000000 ) ) ;
#9071=DIRECTION ( 'NONE',  ( -0.5394184268574406804, 0.8420378618367728718, 0.000000000000000000 ) ) ;
#9078=EDGE_CURVE ( 'NONE', #11277, #8918, #6557, .T. ) ;
#9093=TOROIDAL_SURFACE ( 'NONE', #4924, 1.000000000000000000, 0.5000000000000000000 ) ;
#9095=ORIENTED_EDGE ( 'NONE', *, *, #12039, .T. ) ;
#9105=DIRECTION ( 'NONE',  ( -0.8420378618367728718, -0.5394184268574404584, 0.000000000000000000 ) ) ;
#9106=VECTOR ( 'NONE', #12401, 1000.000000000000000 ) ;
#9110=DIRECTION ( 'NONE',  ( -0.000000000000000000, -0.000000000000000000, -1.000000000000000000 ) ) ;
#9111=VERTEX_POINT ( 'NONE', #785 ) ;
#9113=EDGE_LOOP ( 'NONE', ( #14478, #9248, #5993, #10451 ) ) ;
#9114=LINE ( 'NONE', #6495, #53 ) ;
#9119=DIRECTION ( 'NONE',  ( 1.000000000000000000, 1.789942591005740441E-15, 0.000000000000000000 ) ) ;
#9121=AXIS2_PLACEMENT_3D ( 'NONE', #13515, #7520, #655 ) ;
#9123=EDGE_CURVE ( 'NONE', #2463, #10590, #3913, .T. ) ;
#9124=AXIS2_PLACEMENT_3D ( 'NONE', #1687, #14605, #6452 ) ;
#9129=CARTESIAN_POINT ( 'NONE',  ( -12.33418063572647938, -2.249290599286303927, 50.00000000000012079 ) ) ;
#9132=DIRECTION ( 'NONE',  ( 0.000000000000000000, 0.000000000000000000, -1.000000000000000000 ) ) ;
#9137=DIRECTION ( 'NONE',  ( 1.000000000000000000, 0.000000000000000000, 0.000000000000000000 ) ) ;
#9139=ORIENTED_EDGE ( 'NONE', *, *, #641, .T. ) ;
#9141=DIRECTION ( 'NONE',  ( 0.5006040828730246028, -0.8656763553493059815, 0.000000000000000000 ) ) ;
#9149=EDGE_CURVE ( 'NONE', #4049, #5382, #4148, .T. ) ;
#9151=EDGE_CURVE ( 'NONE', #7221, #56, #5390, .T. ) ;
#9159=DIRECTION ( 'NONE',  ( -0.8656763553492972108, -0.5006040828730397019, 1.548731138869852323E-14 ) ) ;
#9166=AXIS2_PLACEMENT_3D ( 'NONE', #12217, #6301, #1748 ) ;
#9168=ORIENTED_EDGE ( 'NONE', *, *, #388, .T. ) ;
#9178=LINE ( 'NONE', #13627, #9106 ) ;
#9179=ORIENTED_EDGE ( 'NONE', *, *, #5426, .F. ) ;
#9182=CARTESIAN_POINT ( 'NONE',  ( -9.271822474830662131, -6.861803161813125662, -47.50000000000012079 ) ) ;
#9184=EDGE_LOOP ( 'NONE', ( #7696, #4178, #13295, #15207 ) ) ;
#9201=ORIENTED_EDGE ( 'NONE', *, *, #7671, .F. ) ;
#9208=ADVANCED_FACE ( 'NONE', ( #12959 ), #15034, .F. ) ;
#9210=CARTESIAN_POINT ( 'NONE',  ( -22.45192840590307881, 4.946501455397934954, -48.38495513066926890 ) ) ;
#9222=ORIENTED_EDGE ( 'NONE', *, *, #4133, .T. ) ;
#9227=CARTESIAN_POINT ( 'NONE',  ( -10.27534025206727186, -8.241935476752797030, 47.97348817130912835 ) ) ;
#9228=EDGE_LOOP ( 'NONE', ( #7642, #14387, #2917, #12284 ) ) ;
#9229=VERTEX_POINT ( 'NONE', #5805 ) ;
#9230=CARTESIAN_POINT ( 'NONE',  ( -3.190546569013415379, 0.8906624217387615339, 48.50000000000012079 ) ) ;
#9235=ADVANCED_FACE ( 'NONE', ( #6867 ), #5889, .T. ) ;
#9238=FACE_OUTER_BOUND ( 'NONE', #3826, .T. ) ;
#9239=DIRECTION ( 'NONE',  ( 0.8420378618367728718, 0.5394184268574404584, 0.000000000000000000 ) ) ;
#9246=CARTESIAN_POINT ( 'NONE',  ( -30.80945343098651890, -5.389243620311580329, 48.50000000000012079 ) ) ;
#9248=ORIENTED_EDGE ( 'NONE', *, *, #5484, .T. ) ;
#9253=CARTESIAN_POINT ( 'NONE',  ( -9.619661834299611414, -7.413097564672500361, -47.90685900409895481 ) ) ;
#9254=DIRECTION ( 'NONE',  ( 0.8381289428352243220, 0.5454721580263371949, 0.000000000000000000 ) ) ;
#9256=DIRECTION ( 'NONE',  ( -0.5125013958363124900, -0.8586863916854809986, 0.000000000000000000 ) ) ;
#9264=CIRCLE ( 'NONE', #9766, 0.5000000000000004441 ) ;
#9265=ORIENTED_EDGE ( 'NONE', *, *, #2587, .T. ) ;
#9268=ORIENTED_EDGE ( 'NONE', *, *, #9339, .F. ) ;
#9271=AXIS2_PLACEMENT_3D ( 'NONE', #13267, #345, #3797 ) ;
#9273=LINE ( 'NONE', #12178, #1640 ) ;
#9276=EDGE_CURVE ( 'NONE', #8405, #2288, #11134, .T. ) ;
#9281=CARTESIAN_POINT ( 'NONE',  ( -28.95977857253349796, -8.587818791446737876, -48.00000000000012079 ) ) ;
#9294=VECTOR ( 'NONE', #7141, 1000.000000000000000 ) ;
#9297=DIRECTION ( 'NONE',  ( 0.000000000000000000, 0.000000000000000000, -1.000000000000000000 ) ) ;
#9298=AXIS2_PLACEMENT_3D ( 'NONE', #3254, #12645, #8106 ) ;
#9299=ORIENTED_EDGE ( 'NONE', *, *, #14963, .F. ) ;
#9306=ORIENTED_EDGE ( 'NONE', *, *, #13741, .F. ) ;
#9311=DIRECTION ( 'NONE',  ( 0.000000000000000000, 0.000000000000000000, -1.000000000000000000 ) ) ;
#9312=DIRECTION ( 'NONE',  ( -0.5006040828730974335, 0.8656763553492640151, 0.000000000000000000 ) ) ;
#9313=CARTESIAN_POINT ( 'NONE',  ( -25.46282903980762669, -6.565599745187292946, -48.00000000000012079 ) ) ;
#9319=CARTESIAN_POINT ( 'NONE',  ( -16.99999999999998579, -2.249290599286303927, 50.50000000000012079 ) ) ;
#9332=FACE_OUTER_BOUND ( 'NONE', #3527, .T. ) ;
#9333=ORIENTED_EDGE ( 'NONE', *, *, #2957, .T. ) ;
#9334=CARTESIAN_POINT ( 'NONE',  ( -3.190546569013415379, 0.8906624217387615339, -58.00000000000012079 ) ) ;
#9337=DIRECTION ( 'NONE',  ( -0.8420378618367644341, -0.5394184268574535590, -0.000000000000000000 ) ) ;
#9339=EDGE_CURVE ( 'NONE', #8826, #922, #4657, .T. ) ;
#9354=AXIS2_PLACEMENT_3D ( 'NONE', #10137, #14823, #4273 ) ;
#9358=CARTESIAN_POINT ( 'NONE',  ( -24.80875755767168300, -6.748058119754043460, 48.36238429206898815 ) ) ;
#9366=ORIENTED_EDGE ( 'NONE', *, *, #2292, .T. ) ;
#9384=AXIS2_PLACEMENT_3D ( 'NONE', #2173, #5731, #13032 ) ;
#9385=EDGE_CURVE ( 'NONE', #1961, #7020, #5639, .T. ) ;
#9387=ORIENTED_EDGE ( 'NONE', *, *, #3670, .T. ) ;
#9390=ORIENTED_EDGE ( 'NONE', *, *, #901, .F. ) ;
#9394=VECTOR ( 'NONE', #10811, 1000.000000000000000 ) ;
#9395=PLANE ( 'NONE',  #11335 ) ;
#9397=ORIENTED_EDGE ( 'NONE', *, *, #7632, .T. ) ;
#9401=PLANE ( 'NONE',  #10574 ) ;
#9408=CARTESIAN_POINT ( 'NONE',  ( -16.99999999999998579, -2.249290599286303927, -38.50000000000012790 ) ) ;
#9409=CARTESIAN_POINT ( 'NONE',  ( -16.99999999999998579, -2.249290599286303927, 48.00000000000012079 ) ) ;
#9417=B_SPLINE_CURVE_WITH_KNOTS ( 'NONE', 3,
 ( #13897, #2114, #5433, #5670, #12753, #2277 ),
 .UNSPECIFIED., .F., .F.,
 ( 4, 2, 4 ),
 ( 0.000000000000000000, 0.0003908577252344191651, 0.0007817154504688383302 ),
 .UNSPECIFIED. ) ;
#9419=CARTESIAN_POINT ( 'NONE',  ( -16.99999999999998579, -2.249290599286303927, 57.50000000000012079 ) ) ;
#9421=CARTESIAN_POINT ( 'NONE',  ( -24.64146379341137560, -7.004861575982634037, -47.89606589046130125 ) ) ;
#9423=DIRECTION ( 'NONE',  ( 0.8656763553493062036, 0.5006040828730242698, 0.000000000000000000 ) ) ;
#9433=CARTESIAN_POINT ( 'NONE',  ( -3.190546569013415379, 0.8906624217387615339, 57.50000000000012079 ) ) ;
#9434=CIRCLE ( 'NONE', #2790, 4.665819364273509073 ) ;
#9439=LINE ( 'NONE', #13127, #203 ) ;
#9457=B_SPLINE_CURVE_WITH_KNOTS ( 'NONE', 3,
 ( #7659, #7506, #5050, #14727, #8516, #14443, #2736, #3889 ),
 .UNSPECIFIED., .F., .F.,
 ( 4, 2, 2, 4 ),
 ( 5.262391672463365372E-17, 0.001077686929059507720, 0.002155373858118960796, 0.004310747716237871285 ),
 .UNSPECIFIED. ) ;
#9460=ORIENTED_EDGE ( 'NONE', *, *, #12243, .T. ) ;
#9461=CARTESIAN_POINT ( 'NONE',  ( -24.96222495693456978, -7.431276100536581275, -57.50000000000012079 ) ) ;
#9474=ADVANCED_FACE ( 'NONE', ( #4239 ), #11467, .T. ) ;
#9475=CARTESIAN_POINT ( 'NONE',  ( -16.99999999999998579, -2.249290599286303927, 50.50000000000012079 ) ) ;
#9476=CARTESIAN_POINT ( 'NONE',  ( -9.456839514482961562, 2.659958822950721391, -48.37147253714708484 ) ) ;
#9484=( LENGTH_UNIT ( ) NAMED_UNIT ( * ) SI_UNIT ( .MILLI., .METRE. ) );
#9487=ORIENTED_EDGE ( 'NONE', *, *, #2930, .F. ) ;
#9489=CARTESIAN_POINT ( 'NONE',  ( -3.190546569013415379, 0.8906624217387615339, -48.50000000000012079 ) ) ;
#9498=ORIENTED_EDGE ( 'NONE', *, *, #8304, .F. ) ;
#9500=CARTESIAN_POINT ( 'NONE',  ( -30.80945343098651890, -5.389243620311580329, -48.00000000000012079 ) ) ;
#9502=ORIENTED_EDGE ( 'NONE', *, *, #13363, .T. ) ;
#9506=CARTESIAN_POINT ( 'NONE',  ( -16.99999999999998579, -2.249290599286303927, -47.50000000000012079 ) ) ;
#9509=AXIS2_PLACEMENT_3D ( 'NONE', #10369, #12673, #9141 ) ;
#9512=CARTESIAN_POINT ( 'NONE',  ( -24.54316049702162772, -7.158540003846257882, 48.36906329404664007 ) ) ;
#9517=( GEOMETRIC_REPRESENTATION_CONTEXT ( 3 ) GLOBAL_UNCERTAINTY_ASSIGNED_CONTEXT ( ( #15209 ) ) GLOBAL_UNIT_ASSIGNED_CONTEXT ( ( #9484, #103, #15176 ) ) REPRESENTATION_CONTEXT ( 'NONE', 'WORKASPACE' ) );
#9530=EDGE_CURVE ( 'NONE', #10346, #7613, #5950, .T. ) ;
#9532=VERTEX_POINT ( 'NONE', #12798 ) ;
#9541=ADVANCED_FACE ( 'NONE', ( #4708 ), #5570, .T. ) ;
#9554=ORIENTED_EDGE ( 'NONE', *, *, #4794, .T. ) ;
#9560=CARTESIAN_POINT ( 'NONE',  ( -9.041069614211208361, 1.954516911250973932, -47.50000000000011369 ) ) ;
#9561=DIRECTION ( 'NONE',  ( 1.000000000000000000, 0.000000000000000000, 0.000000000000000000 ) ) ;
#9562=CIRCLE ( 'NONE', #5367, 4.000000000000000000 ) ;
#9563=ORIENTED_EDGE ( 'NONE', *, *, #3488, .T. ) ;
#9564=CARTESIAN_POINT ( 'NONE',  ( -22.95637227168126770, 4.533106128208347130, 48.03392779025640635 ) ) ;
#9565=EDGE_CURVE ( 'NONE', #6058, #8849, #5819, .T. ) ;
#9567=EDGE_CURVE ( 'NONE', #505, #12008, #4067, .T. ) ;
#9569=CARTESIAN_POINT ( 'NONE',  ( -21.85476584171713199, 5.329050157244537900, -48.00000000000012079 ) ) ;
#9573=CARTESIAN_POINT ( 'NONE',  ( -12.14523415828302078, -9.827631355817260328, -48.50000000000012079 ) ) ;
#9575=CARTESIAN_POINT ( 'NONE',  ( -9.107478285483566083, 2.086796655788927701, -48.09696226170978406 ) ) ;
#9584=VERTEX_POINT ( 'NONE', #14745 ) ;
#9592=DIRECTION ( 'NONE',  ( -1.000000000000000000, 0.000000000000000000, 0.000000000000000000 ) ) ;
#9596=CARTESIAN_POINT ( 'NONE',  ( -25.21252699939434194, -6.998437923453657561, 48.43453164808065736 ) ) ;
#9599=CARTESIAN_POINT ( 'NONE',  ( -1.197457146693684082, -2.220571218158921223, -58.00000000000012079 ) ) ;
#9605=ORIENTED_EDGE ( 'NONE', *, *, #9385, .F. ) ;
#9612=CARTESIAN_POINT ( 'NONE',  ( -25.15752072101212278, 2.619472661158555038, 48.00000000000012079 ) ) ;
#9614=EDGE_CURVE ( 'NONE', #3355, #3566, #8486, .T. ) ;
#9616=EDGE_CURVE ( 'NONE', #12776, #7020, #5076, .T. ) ;
#9620=CARTESIAN_POINT ( 'NONE',  ( -12.99999999999998757, -2.249290599286303927, 38.00000000000012079 ) ) ;
#9623=CIRCLE ( 'NONE', #8094, 8.500000000000000000 ) ;
#9626=CARTESIAN_POINT ( 'NONE',  ( -10.08762850755046969, -8.023634329963208245, 47.66527511103321046 ) ) ;
#9638=DIRECTION ( 'NONE',  ( 0.8908241094534407045, 0.4543483311474627029, 0.000000000000000000 ) ) ;
#9642=ORIENTED_EDGE ( 'NONE', *, *, #9151, .T. ) ;
#9651=CARTESIAN_POINT ( 'NONE',  ( -9.148597373295839219, 2.167486929505451076, -48.18452149279841024 ) ) ;
#9652=FACE_OUTER_BOUND ( 'NONE', #13673, .T. ) ;
#9668=DIRECTION ( 'NONE',  ( -0.000000000000000000, -0.000000000000000000, -1.000000000000000000 ) ) ;
#9669=AXIS2_PLACEMENT_3D ( 'NONE', #12801, #856, #10254 ) ;
#9672=AXIS2_PLACEMENT_3D ( 'NONE', #5200, #11901, #14584 ) ;
#9686=ORIENTED_EDGE ( 'NONE', *, *, #13099, .F. ) ;
#9688=DIRECTION ( 'NONE',  ( 0.5394184268574520047, -0.8420378618367654333, 0.000000000000000000 ) ) ;
#9707=DIRECTION ( 'NONE',  ( -0.5006040828730976555, 0.8656763553492637930, 0.000000000000000000 ) ) ;
#9716=DIRECTION ( 'NONE',  ( 0.000000000000000000, -0.000000000000000000, -1.000000000000000000 ) ) ;
#9718=CARTESIAN_POINT ( 'NONE',  ( -22.42998452855183444, 4.960558937058127782, 48.26605223428308733 ) ) ;
#9729=DIRECTION ( 'NONE',  ( -0.000000000000000000, -0.000000000000000000, -1.000000000000000000 ) ) ;
#9732=EDGE_CURVE ( 'NONE', #4371, #3752, #10294, .T. ) ;
#9734=CARTESIAN_POINT ( 'NONE',  ( -16.99999999999998579, -2.249290599286303927, -50.00000000000012079 ) ) ;
#9747=ORIENTED_EDGE ( 'NONE', *, *, #12708, .T. ) ;
#9758=AXIS2_PLACEMENT_3D ( 'NONE', #6512, #13670, #5214 ) ;
#9759=CARTESIAN_POINT ( 'NONE',  ( -22.16581936427349575, -2.249290599286304371, -57.50000000000012079 ) ) ;
#9760=ORIENTED_EDGE ( 'NONE', *, *, #6868, .T. ) ;
#9761=DIRECTION ( 'NONE',  ( 1.000000000000000000, 0.000000000000000000, 0.000000000000000000 ) ) ;
#9766=AXIS2_PLACEMENT_3D ( 'NONE', #6283, #10974, #429 ) ;
#9769=CARTESIAN_POINT ( 'NONE',  ( -21.99701278316016584, 5.237925250804929433, 48.44214661496815211 ) ) ;
#9772=EDGE_CURVE ( 'NONE', #4994, #7307, #888, .T. ) ;
#9776=DIRECTION ( 'NONE',  ( 1.000000000000000000, -2.602085213965208275E-15, 0.000000000000000000 ) ) ;
#9777=FACE_OUTER_BOUND ( 'NONE', #4330, .T. ) ;
#9780=ORIENTED_EDGE ( 'NONE', *, *, #7759, .T. ) ;
#9787=CARTESIAN_POINT ( 'NONE',  ( -23.95855436784179560, 3.468451880982295954, 47.93156476714377590 ) ) ;
#9792=FACE_OUTER_BOUND ( 'NONE', #5654, .T. ) ;
#9797=DIRECTION ( 'NONE',  ( 1.000000000000000000, 0.000000000000000000, 0.000000000000000000 ) ) ;
#9798=AXIS2_PLACEMENT_3D ( 'NONE', #11625, #1081, #5792 ) ;
#9811=CARTESIAN_POINT ( 'NONE',  ( -9.084028622109864060, 2.040253803610913685, 48.06338840812200175 ) ) ;
#9813=CARTESIAN_POINT ( 'NONE',  ( -24.55590860040002710, -7.139109479066534369, -48.24517880332174968 ) ) ;
#9814=DIRECTION ( 'NONE',  ( -0.000000000000000000, 0.000000000000000000, 1.000000000000000000 ) ) ;
#9820=DIRECTION ( 'NONE',  ( 1.000000000000000000, 0.000000000000000000, 0.000000000000000000 ) ) ;
#9822=ORIENTED_EDGE ( 'NONE', *, *, #7544, .F. ) ;
#9826=DIRECTION ( 'NONE',  ( 0.000000000000000000, 0.000000000000000000, -1.000000000000000000 ) ) ;
#9829=DIRECTION ( 'NONE',  ( 1.000000000000000000, 0.000000000000000000, 0.000000000000000000 ) ) ;
#9837=EDGE_CURVE ( 'NONE', #1708, #9017, #3112, .T. ) ;
#9850=EDGE_LOOP ( 'NONE', ( #2494, #8153, #12047, #13823 ) ) ;
#9853=ORIENTED_EDGE ( 'NONE', *, *, #5612, .T. ) ;
#9856=DIRECTION ( 'NONE',  ( -0.000000000000000000, 0.000000000000000000, 1.000000000000000000 ) ) ;
#9860=EDGE_LOOP ( 'NONE', ( #11905, #12817, #9760, #13945 ) ) ;
#9873=CARTESIAN_POINT ( 'NONE',  ( -9.871163676013017252, -8.117995983050501962, -48.08465436988272046 ) ) ;
#9880=ORIENTED_EDGE ( 'NONE', *, *, #1566, .F. ) ;
#9883=AXIS2_PLACEMENT_3D ( 'NONE', #3166, #7716, #12403 ) ;
#9885=AXIS2_PLACEMENT_3D ( 'NONE', #8682, #12375, #14531 ) ;
#9898=AXIS2_PLACEMENT_3D ( 'NONE', #8542, #13242, #2687 ) ;
#9903=AXIS2_PLACEMENT_3D ( 'NONE', #3687, #4921, #9311 ) ;
#9911=VERTEX_POINT ( 'NONE', #2440 ) ;
#9912=ORIENTED_EDGE ( 'NONE', *, *, #6225, .F. ) ;
#9920=EDGE_LOOP ( 'NONE', ( #1712, #11182, #13075, #9095 ) ) ;
#9921=AXIS2_PLACEMENT_3D ( 'NONE', #290, #6226, #3674 ) ;
#9923=CARTESIAN_POINT ( 'NONE',  ( -3.535822565187055400, 6.114368811827579187, 57.50000000000012079 ) ) ;
#9924=ORIENTED_EDGE ( 'NONE', *, *, #10546, .F. ) ;
#9926=AXIS2_PLACEMENT_3D ( 'NONE', #5377, #13608, #2773 ) ;
#9927=DIRECTION ( 'NONE',  ( 0.8420378618367644341, 0.5394184268574535590, 0.000000000000000000 ) ) ;
#9937=ORIENTED_EDGE ( 'NONE', *, *, #5554, .T. ) ;
#9943=EDGE_CURVE ( 'NONE', #5460, #12879, #2626, .T. ) ;
#9944=DIRECTION ( 'NONE',  ( 0.8656763553492639041, 0.5006040828730973224, -0.000000000000000000 ) ) ;
#9948=LINE ( 'NONE', #1922, #4499 ) ;
#9950=ORIENTED_EDGE ( 'NONE', *, *, #6357, .T. ) ;
#9952=CARTESIAN_POINT ( 'NONE',  ( -8.650962968042231083, 2.291620771759304898, 48.06291368403883268 ) ) ;
#9957=CARTESIAN_POINT ( 'NONE',  ( -16.99999999999998579, -2.249290599286303927, 57.50000000000012079 ) ) ;
#9974=EDGE_CURVE ( 'NONE', #7994, #355, #3360, .T. ) ;
#9978=ORIENTED_EDGE ( 'NONE', *, *, #6408, .T. ) ;
#9980=ORIENTED_EDGE ( 'NONE', *, *, #2725, .F. ) ;
#9989=EDGE_LOOP ( 'NONE', ( #1553, #9062, #6070, #12671 ) ) ;
#9991=EDGE_LOOP ( 'NONE', ( #8382, #1357, #5270, #11558 ) ) ;
#9995=CARTESIAN_POINT ( 'NONE',  ( -30.80945343098651890, -5.389243620311580329, 48.50000000000012079 ) ) ;
#9997=FACE_OUTER_BOUND ( 'NONE', #4663, .T. ) ;
#9998=ORIENTED_EDGE ( 'NONE', *, *, #2793, .T. ) ;
#10004=ORIENTED_EDGE ( 'NONE', *, *, #12463, .F. ) ;
#10006=VECTOR ( 'NONE', #10809, 1000.000000000000000 ) ;
#10009=DIRECTION ( 'NONE',  ( 1.000000000000000000, 0.000000000000000000, 0.000000000000000000 ) ) ;
#10010=ORIENTED_EDGE ( 'NONE', *, *, #1124, .T. ) ;
#10015=AXIS2_PLACEMENT_3D ( 'NONE', #2388, #8167, #8328 ) ;
#10016=DIRECTION ( 'NONE',  ( -0.000000000000000000, -0.000000000000000000, -1.000000000000000000 ) ) ;
#10019=AXIS2_PLACEMENT_3D ( 'NONE', #6860, #3091, #10180 ) ;
#10024=ORIENTED_EDGE ( 'NONE', *, *, #12051, .F. ) ;
#10028=FACE_OUTER_BOUND ( 'NONE', #1770, .T. ) ;
#10029=AXIS2_PLACEMENT_3D ( 'NONE', #13874, #4483, #7874 ) ;
#10033=CARTESIAN_POINT ( 'NONE',  ( -25.43628086306388525, -6.625164433253370788, -48.00000000000012079 ) ) ;
#10035=EDGE_CURVE ( 'NONE', #15152, #864, #11462, .T. ) ;
#10036=ADVANCED_FACE ( 'NONE', ( #1871, #4106 ), #499, .T. ) ;
#10043=EDGE_LOOP ( 'NONE', ( #9139, #2910, #9306, #10024 ) ) ;
#10058=AXIS2_PLACEMENT_3D ( 'NONE', #1637, #2946, #13337 ) ;
#10063=CARTESIAN_POINT ( 'NONE',  ( -9.037775043065352065, 2.932694901963889489, -58.00000000000012079 ) ) ;
#10067=ADVANCED_FACE ( 'NONE', ( #13355 ), #4029, .T. ) ;
#10069=EDGE_CURVE ( 'NONE', #10590, #298, #8030, .T. ) ;
#10075=DIRECTION ( 'NONE',  ( 0.000000000000000000, 0.000000000000000000, -1.000000000000000000 ) ) ;
#10081=AXIS2_PLACEMENT_3D ( 'NONE', #10524, #2286, #5677 ) ;
#10084=CARTESIAN_POINT ( 'NONE',  ( -24.14404371603619381, 3.605862562765568491, -48.08251050686933326 ) ) ;
#10095=CARTESIAN_POINT ( 'NONE',  ( -9.009135308666344599, 1.891904487837172910, 48.00342231809197102 ) ) ;
#10096=ORIENTED_EDGE ( 'NONE', *, *, #7671, .T. ) ;
#10099=TOROIDAL_SURFACE ( 'NONE', #2971, 3.694885682587998765, 0.5000000000000000000 ) ;
#10100=DIRECTION ( 'NONE',  ( 1.000000000000000000, 0.000000000000000000, 0.000000000000000000 ) ) ;
#10104=EDGE_CURVE ( 'NONE', #12776, #6801, #11120, .T. ) ;
#10106=EDGE_CURVE ( 'NONE', #5460, #170, #9264, .T. ) ;
#10112=CYLINDRICAL_SURFACE ( 'NONE', #2206, 4.000000000000000000 ) ;
#10130=CIRCLE ( 'NONE', #12103, 0.4999999999999999445 ) ;
#10137=CARTESIAN_POINT ( 'NONE',  ( -1.197457146693683194, -2.220571218158922999, 57.50000000000012079 ) ) ;
#10141=CARTESIAN_POINT ( 'NONE',  ( -3.190546569013415379, 0.8906624217387615339, -58.00000000000012079 ) ) ;
#10149=DIRECTION ( 'NONE',  ( 0.8420378618367644341, 0.5394184268574535590, 0.000000000000000000 ) ) ;
#10150=ORIENTED_EDGE ( 'NONE', *, *, #7246, .F. ) ;
#10152=CARTESIAN_POINT ( 'NONE',  ( -16.99999999999998579, -2.249290599286303927, 38.50000000000012790 ) ) ;
#10161=CARTESIAN_POINT ( 'NONE',  ( -24.54301448188264700, 2.673459138797629198, -47.50000001881890910 ) ) ;
#10166=CARTESIAN_POINT ( 'NONE',  ( -24.96222495693456978, -7.431276100536581275, 57.50000000000012079 ) ) ;
#10167=ADVANCED_FACE ( 'NONE', ( #4498 ), #13733, .T. ) ;
#10168=CARTESIAN_POINT ( 'NONE',  ( -9.456839514482961562, 2.659958822950721391, 48.37147253714708484 ) ) ;
#10170=VECTOR ( 'NONE', #11428, 1000.000000000000000 ) ;
#10177=( LENGTH_UNIT ( ) NAMED_UNIT ( * ) SI_UNIT ( .MILLI., .METRE. ) );
#10178=DIRECTION ( 'NONE',  ( 0.5006040828730989878, -0.8656763553492631269, 0.000000000000000000 ) ) ;
#10180=DIRECTION ( 'NONE',  ( 1.000000000000000000, 0.000000000000000000, 0.000000000000000000 ) ) ;
#10187=CARTESIAN_POINT ( 'NONE',  ( -24.96151347116557062, -6.448033549061094938, -47.50000000626571506 ) ) ;
#10188=ORIENTED_EDGE ( 'NONE', *, *, #8257, .T. ) ;
#10192=ORIENTED_EDGE ( 'NONE', *, *, #974, .F. ) ;
#10199=DIRECTION ( 'NONE',  ( 1.000000000000000000, 3.565820478396769525E-15, 0.000000000000000000 ) ) ;
#10204=VERTEX_POINT ( 'NONE', #6726 ) ;
#10213=CARTESIAN_POINT ( 'NONE',  ( -16.99999999999998579, -2.249290599286303927, 47.50000000000012079 ) ) ;
#10217=CARTESIAN_POINT ( 'NONE',  ( -25.21252699837112132, -6.998437922861946880, 58.00000000000012079 ) ) ;
#10227=CYLINDRICAL_SURFACE ( 'NONE', #6684, 4.194885682588113340 ) ;
#10231=CARTESIAN_POINT ( 'NONE',  ( -23.91311688008704905, 3.524160940036151324, -47.66502101098827637 ) ) ;
#10236=VERTEX_POINT ( 'NONE', #10432 ) ;
#10239=CARTESIAN_POINT ( 'NONE',  ( -7.999999999999986677, -2.249290599286302594, 58.00000000000012079 ) ) ;
#10243=CARTESIAN_POINT ( 'NONE',  ( -5.040221427466046400, 4.089237592873870675, 48.50000000000012079 ) ) ;
#10246=LINE ( 'NONE', #14939, #7385 ) ;
#10254=DIRECTION ( 'NONE',  ( 0.000000000000000000, 0.000000000000000000, -1.000000000000000000 ) ) ;
#10257=CARTESIAN_POINT ( 'NONE',  ( -8.787473001628836045, 2.499856724289236887, -48.50000000000012079 ) ) ;
#10258=AXIS2_PLACEMENT_3D ( 'NONE', #6886, #7891, #10199 ) ;
#10266=AXIS2_PLACEMENT_3D ( 'NONE', #12925, #11828, #7067 ) ;
#10276=CARTESIAN_POINT ( 'NONE',  ( -30.80945343098651890, -5.389243620311580329, 48.00000000000012079 ) ) ;
#10284=FACE_OUTER_BOUND ( 'NONE', #5421, .T. ) ;
#10288=ORIENTED_EDGE ( 'NONE', *, *, #11053, .F. ) ;
#10292=VERTEX_POINT ( 'NONE', #8119 ) ;
#10294=LINE ( 'NONE', #13986, #14179 ) ;
#10299=ADVANCED_FACE ( 'NONE', ( #12819 ), #3503, .F. ) ;
#10302=CARTESIAN_POINT ( 'NONE',  ( -16.99999999999998579, -2.249290599286303927, 57.50000000000012079 ) ) ;
#10303=CARTESIAN_POINT ( 'NONE',  ( -12.14523415828302078, -9.827631355817260328, 48.50000000000012079 ) ) ;
#10305=DIRECTION ( 'NONE',  ( 1.000000000000000000, 0.000000000000000000, 0.000000000000000000 ) ) ;
#10309=DIRECTION ( 'NONE',  ( 0.000000000000000000, 0.000000000000000000, -1.000000000000000000 ) ) ;
#10310=CARTESIAN_POINT ( 'NONE',  ( -21.85476584171706449, 5.329050157244580532, -48.50000000000012079 ) ) ;
#10319=DIRECTION ( 'NONE',  ( 0.8656763553492639041, 0.5006040828730973224, -0.000000000000000000 ) ) ;
#10325=DIRECTION ( 'NONE',  ( 0.000000000000000000, 0.000000000000000000, -1.000000000000000000 ) ) ;
#10327=DIRECTION ( 'NONE',  ( 0.000000000000000000, 0.000000000000000000, -1.000000000000000000 ) ) ;
#10330=CARTESIAN_POINT ( 'NONE',  ( -9.271822474830681671, -6.861803161813159413, -48.00000000000019895 ) ) ;
#10332=EDGE_LOOP ( 'NONE', ( #7926, #14712, #12796, #3951 ) ) ;
#10335=AXIS2_PLACEMENT_3D ( 'NONE', #11091, #4010, #7488 ) ;
#10341=CIRCLE ( 'NONE', #13530, 9.000000000000001776 ) ;
#10346=VERTEX_POINT ( 'NONE', #10889 ) ;
#10350=TOROIDAL_SURFACE ( 'NONE', #12310, 4.165819364273509962, 0.5000000000000000000 ) ;
#10352=VECTOR ( 'NONE', #14093, 1000.000000000000000 ) ;
#10354=DIRECTION ( 'NONE',  ( 1.000000000000000000, 0.000000000000000000, 0.000000000000000000 ) ) ;
#10359=ORIENTED_EDGE ( 'NONE', *, *, #707, .F. ) ;
#10360=EDGE_CURVE ( 'NONE', #7307, #7221, #13694, .T. ) ;
#10364=ORIENTED_EDGE ( 'NONE', *, *, #8857, .T. ) ;
#10367=ORIENTED_EDGE ( 'NONE', *, *, #9837, .T. ) ;
#10369=CARTESIAN_POINT ( 'NONE',  ( -5.040221427466112125, 4.089237592873837812, 57.50000000000012079 ) ) ;
#10370=ADVANCED_FACE ( 'NONE', ( #4887 ), #7064, .F. ) ;
#10379=CARTESIAN_POINT ( 'NONE',  ( -12.14523415828302078, -9.827631355817260328, 48.50000000000012079 ) ) ;
#10380=EDGE_LOOP ( 'NONE', ( #7149, #6038, #11924, #3980 ) ) ;
#10384=DIRECTION ( 'NONE',  ( -0.8420378618367727608, -0.5394184268574406804, -0.000000000000000000 ) ) ;
#10385=ORIENTED_EDGE ( 'NONE', *, *, #1335, .T. ) ;
#10388=EDGE_CURVE ( 'NONE', #13060, #3246, #14920, .T. ) ;
#10392=CARTESIAN_POINT ( 'NONE',  ( -24.57377864815406099, 2.621914368698142983, -47.92899112040971943 ) ) ;
#10394=CARTESIAN_POINT ( 'NONE',  ( -12.14523415828296216, -9.827631355817223024, 48.50000000000012079 ) ) ;
#10410=EDGE_CURVE ( 'NONE', #13060, #7307, #11729, .T. ) ;
#10421=DIRECTION ( 'NONE',  ( 0.000000000000000000, -0.000000000000000000, -1.000000000000000000 ) ) ;
#10422=CARTESIAN_POINT ( 'NONE',  ( -5.040221427466109461, 4.089237592873834259, 48.00000000000012079 ) ) ;
#10425=EDGE_CURVE ( 'NONE', #14061, #6293, #9023, .T. ) ;
#10432=CARTESIAN_POINT ( 'NONE',  ( -24.72817752516938228, 2.363221963240404566, 47.50000000000012079 ) ) ;
#10434=CARTESIAN_POINT ( 'NONE',  ( -12.83418063572647760, -2.249290599286303927, 50.00000000000012079 ) ) ;
#10436=DIRECTION ( 'NONE',  ( -0.000000000000000000, -0.000000000000000000, 1.000000000000000000 ) ) ;
#10451=ORIENTED_EDGE ( 'NONE', *, *, #6045, .T. ) ;
#10452=DIRECTION ( 'NONE',  ( 0.000000000000000000, 0.000000000000000000, -1.000000000000000000 ) ) ;
#10455=CARTESIAN_POINT ( 'NONE',  ( -11.53791661996513085, -9.438577269332638409, 48.38299871084047510 ) ) ;
#10470=VECTOR ( 'NONE', #9944, 1000.000000000000114 ) ;
#10482=CARTESIAN_POINT ( 'NONE',  ( -10.27534025206727186, -8.241935476752797030, -47.97348817130912835 ) ) ;
#10483=DIRECTION ( 'NONE',  ( -0.8656763553492639041, -0.5006040828730973224, -0.000000000000000000 ) ) ;
#10494=DIRECTION ( 'NONE',  ( -0.000000000000000000, 0.000000000000000000, 1.000000000000000000 ) ) ;
#10495=ORIENTED_EDGE ( 'NONE', *, *, #5807, .F. ) ;
#10499=CIRCLE ( 'NONE', #1152, 0.5000000000000004441 ) ;
#10503=CIRCLE ( 'NONE', #9271, 4.194885682588113340 ) ;
#10510=ADVANCED_FACE ( 'NONE', ( #5260 ), #5843, .T. ) ;
#10522=CARTESIAN_POINT ( 'NONE',  ( -5.290523468902621929, 4.522075770548486418, 48.50000000000012079 ) ) ;
#10524=CARTESIAN_POINT ( 'NONE',  ( -16.99999999999998579, -2.249290599286303927, 47.50000000000012079 ) ) ;
#10530=AXIS2_PLACEMENT_3D ( 'NONE', #2914, #2483, #4795 ) ;
#10531=EDGE_LOOP ( 'NONE', ( #9201, #10825, #7002, #11565, #7924, #8204, #9937, #5146, #12125, #2138, #11237 ) ) ;
#10537=ORIENTED_EDGE ( 'NONE', *, *, #503, .T. ) ;
#10538=LINE ( 'NONE', #14911, #15166 ) ;
#10539=ORIENTED_EDGE ( 'NONE', *, *, #4423, .T. ) ;
#10541=EDGE_LOOP ( 'NONE', ( #353, #5848 ) ) ;
#10546=EDGE_CURVE ( 'NONE', #6843, #60, #8306, .T. ) ;
#10549=CARTESIAN_POINT ( 'NONE',  ( -8.537170960192302260, 2.067018546614596719, 48.00000000000012079 ) ) ;
#10559=EDGE_LOOP ( 'NONE', ( #4194, #9366 ) ) ;
#10563=VECTOR ( 'NONE', #13406, 1000.000000000000000 ) ;
#10566=CARTESIAN_POINT ( 'NONE',  ( -11.53791661996513085, -9.438577269332638409, -48.38299871084047510 ) ) ;
#10567=DIRECTION ( 'NONE',  ( -0.000000000000000000, -0.000000000000000000, 1.000000000000000000 ) ) ;
#10573=CARTESIAN_POINT ( 'NONE',  ( -24.78493442214762155, -6.766828585132234508, -47.63220435834860922 ) ) ;
#10574=AXIS2_PLACEMENT_3D ( 'NONE', #4702, #9063, #896 ) ;
#10586=CARTESIAN_POINT ( 'NONE',  ( -16.99999999999998579, -2.249290599286303927, 38.00000000000012079 ) ) ;
#10587=CARTESIAN_POINT ( 'NONE',  ( -25.34903703195771385, -6.790201970332132575, 48.06291368403887532 ) ) ;
#10590=VERTEX_POINT ( 'NONE', #12332 ) ;
#10595=ORIENTED_EDGE ( 'NONE', *, *, #14963, .T. ) ;
#10602=ORIENTED_EDGE ( 'NONE', *, *, #10106, .F. ) ;
#10604=CARTESIAN_POINT ( 'NONE',  ( -21.85476584171713199, 5.329050157244537900, 48.50000000000012079 ) ) ;
#10616=CARTESIAN_POINT ( 'NONE',  ( -23.19801677984724364, 4.285555568094122414, -47.93908580834070676 ) ) ;
#10624=DIRECTION ( 'NONE',  ( 0.5006040828730989878, -0.8656763553492631269, 0.000000000000000000 ) ) ;
#10625=CARTESIAN_POINT ( 'NONE',  ( -9.444091399599896519, 2.640528280493846580, -48.24517880332174968 ) ) ;
#10626=ADVANCED_FACE ( 'NONE', ( #10028 ), #7556, .T. ) ;
#10642=CARTESIAN_POINT ( 'NONE',  ( -9.035163663297472780, 1.943345362497546747, -48.01692658285808335 ) ) ;
#10662=TOROIDAL_SURFACE ( 'NONE', #5249, 3.694885682588112452, 0.5000000000000000000 ) ;
#10665=DIRECTION ( 'NONE',  ( 0.8420378618367644341, 0.5394184268574535590, 0.000000000000000000 ) ) ;
#10668=ADVANCED_FACE ( 'NONE', ( #5798 ), #4103, .T. ) ;
#10676=ORIENTED_EDGE ( 'NONE', *, *, #7759, .F. ) ;
#10678=CARTESIAN_POINT ( 'NONE',  ( -16.99999999999998579, -2.249290599286303927, -38.50000000000012790 ) ) ;
#10685=CYLINDRICAL_SURFACE ( 'NONE', #1409, 9.000000000000001776 ) ;
#10690=ORIENTED_EDGE ( 'NONE', *, *, #9567, .F. ) ;
#10694=EDGE_LOOP ( 'NONE', ( #10367, #2141, #14779, #14136 ) ) ;
#10695=CARTESIAN_POINT ( 'NONE',  ( -24.34228330361342785, 2.967490118658024034, -47.54143911729025973 ) ) ;
#10697=ORIENTED_EDGE ( 'NONE', *, *, #11766, .T. ) ;
#10698=DIRECTION ( 'NONE',  ( -0.8381289428352193260, -0.5454721580263449665, 0.000000000000000000 ) ) ;
#10703=CARTESIAN_POINT ( 'NONE',  ( -24.54316048551696028, -7.158540021523408292, 48.50000000000012079 ) ) ;
#10705=CARTESIAN_POINT ( 'NONE',  ( -16.99999999999998579, -2.249290599286303927, 50.00000000000012079 ) ) ;
#10712=VERTEX_POINT ( 'NONE', #4312 ) ;
#10713=CARTESIAN_POINT ( 'NONE',  ( -12.14523415828302078, -9.827631355817260328, -48.50000000000012079 ) ) ;
#10715=CARTESIAN_POINT ( 'NONE',  ( -9.443282642412393457, 2.639297360524499592, -48.23807154671105479 ) ) ;
#10723=ORIENTED_EDGE ( 'NONE', *, *, #14642, .T. ) ;
#10729=CYLINDRICAL_SURFACE ( 'NONE', #2537, 0.5000000000000000000 ) ;
#10734=CIRCLE ( 'NONE', #15158, 0.5000000000000004441 ) ;
#10737=CARTESIAN_POINT ( 'NONE',  ( -24.96151347116557062, -6.448033549061094938, 47.50000000626571506 ) ) ;
#10738=CIRCLE ( 'NONE', #13201, 4.194885682588113340 ) ;
#10742=DIRECTION ( 'NONE',  ( 0.5006040828730401460, -0.8656763553492970997, 0.000000000000000000 ) ) ;
#10744=EDGE_CURVE ( 'NONE', #5398, #12776, #11394, .T. ) ;
#10747=EDGE_LOOP ( 'NONE', ( #14619, #5556, #14096, #269 ) ) ;
#10762=DIRECTION ( 'NONE',  ( -0.8656763553492639041, -0.5006040828730973224, 0.000000000000000000 ) ) ;
#10767=DIRECTION ( 'NONE',  ( 1.000000000000000000, 0.000000000000000000, 0.000000000000000000 ) ) ;
#10775=DIRECTION ( 'NONE',  ( -0.5454721580263448555, 0.8381289428352193260, 0.000000000000000000 ) ) ;
#10781=CARTESIAN_POINT ( 'NONE',  ( -9.358536206588548012, 2.506280377409947135, -47.89606589046130125 ) ) ;
#10783=AXIS2_PLACEMENT_3D ( 'NONE', #10586, #4659, #3428 ) ;
#10784=EDGE_LOOP ( 'NONE', ( #12496, #4140, #2513, #7292 ) ) ;
#10788=DIRECTION ( 'NONE',  ( 1.000000000000000000, 0.000000000000000000, 0.000000000000000000 ) ) ;
#10790=ADVANCED_FACE ( 'NONE', ( #6943 ), #1462, .F. ) ;
#10797=AXIS2_PLACEMENT_3D ( 'NONE', #1307, #90, #11619 ) ;
#10809=DIRECTION ( 'NONE',  ( 0.8656763553493062036, 0.5006040828730242698, -0.000000000000000000 ) ) ;
#10811=DIRECTION ( 'NONE',  ( -0.8420378618367644341, -0.5394184268574535590, -0.000000000000000000 ) ) ;
#10817=VERTEX_POINT ( 'NONE', #7099 ) ;
#10822=AXIS2_PLACEMENT_3D ( 'NONE', #5291, #7750, #8898 ) ;
#10825=ORIENTED_EDGE ( 'NONE', *, *, #6298, .T. ) ;
#10826=DIRECTION ( 'NONE',  ( -0.000000000000000000, -0.000000000000000000, 1.000000000000000000 ) ) ;
#10833=DIRECTION ( 'NONE',  ( -0.8420378618367728718, -0.5394184268574404584, 0.000000000000000000 ) ) ;
#10835=ORIENTED_EDGE ( 'NONE', *, *, #5807, .T. ) ;
#10838=ORIENTED_EDGE ( 'NONE', *, *, #7752, .F. ) ;
#10850=LINE ( 'NONE', #3464, #2748 ) ;
#10853=VERTEX_POINT ( 'NONE', #13029 ) ;
#10860=EDGE_CURVE ( 'NONE', #13513, #14513, #172, .T. ) ;
#10862=CIRCLE ( 'NONE', #12565, 0.5000000000000001110 ) ;
#10869=CARTESIAN_POINT ( 'NONE',  ( -12.99999999999998757, -2.249290599286303927, -38.00000000000012079 ) ) ;
#10879=CARTESIAN_POINT ( 'NONE',  ( -24.54316048551696383, -7.158540021523408292, 48.37147253714708484 ) ) ;
#10881=CIRCLE ( 'NONE', #9669, 0.5000000000000004441 ) ;
#10883=ADVANCED_FACE ( 'NONE', ( #11016 ), #193, .T. ) ;
#10889=CARTESIAN_POINT ( 'NONE',  ( -21.85476584171713199, 5.329050157244537900, -48.50000000000012079 ) ) ;
#10895=DIRECTION ( 'NONE',  ( 1.000000000000000000, 0.000000000000000000, 0.000000000000000000 ) ) ;
#10911=DIRECTION ( 'NONE',  ( 1.000000000000000000, 0.000000000000000000, 0.000000000000000000 ) ) ;
#10916=DIRECTION ( 'NONE',  ( -1.000000000000000000, 0.000000000000000000, 0.000000000000000000 ) ) ;
#10918=ORIENTED_EDGE ( 'NONE', *, *, #13099, .T. ) ;
#10923=DIRECTION ( 'NONE',  ( 0.000000000000000000, 0.000000000000000000, -1.000000000000000000 ) ) ;
#10925=CARTESIAN_POINT ( 'NONE',  ( -3.190546569013415379, 0.8906624217387615339, -48.50000000000012079 ) ) ;
#10926=VERTEX_POINT ( 'NONE', #13537 ) ;
#10929=LINE ( 'NONE', #452, #11211 ) ;
#10932=CYLINDRICAL_SURFACE ( 'NONE', #8161, 0.4999999999999996669 ) ;
#10938=CARTESIAN_POINT ( 'NONE',  ( -3.190546569013415379, 0.8906624217387615339, 48.00000000000012079 ) ) ;
#10939=ORIENTED_EDGE ( 'NONE', *, *, #7268, .F. ) ;
#10955=CARTESIAN_POINT ( 'NONE',  ( -8.779681704480811533, 2.489320016922789147, 48.36903577193039894 ) ) ;
#10964=DIRECTION ( 'NONE',  ( 0.000000000000000000, 0.000000000000000000, -1.000000000000000000 ) ) ;
#10965=CARTESIAN_POINT ( 'NONE',  ( -25.21252699837112132, -6.998437922861948657, -48.50000000000011369 ) ) ;
#10969=VERTEX_POINT ( 'NONE', #10869 ) ;
#10972=EDGE_LOOP ( 'NONE', ( #3319, #8076, #8450, #12144 ) ) ;
#10974=DIRECTION ( 'NONE',  ( -0.000000000000000000, 1.000000000000000000, 0.000000000000000000 ) ) ;
#10976=AXIS2_PLACEMENT_3D ( 'NONE', #9409, #6940, #10788 ) ;
#10985=AXIS2_PLACEMENT_3D ( 'NONE', #361, #4824, #9688 ) ;
#10987=VERTEX_POINT ( 'NONE', #5700 ) ;
#10999=AXIS2_PLACEMENT_3D ( 'NONE', #9957, #12405, #12179 ) ;
#11003=CARTESIAN_POINT ( 'NONE',  ( -9.271822474830662131, -6.861803161813125662, 47.50000000000012079 ) ) ;
#11011=ORIENTED_EDGE ( 'NONE', *, *, #3727, .F. ) ;
#11016=FACE_OUTER_BOUND ( 'NONE', #2538, .T. ) ;
#11021=CIRCLE ( 'NONE', #10783, 8.500000000000000000 ) ;
#11024=DIRECTION ( 'NONE',  ( 0.000000000000000000, -0.000000000000000000, -1.000000000000000000 ) ) ;
#11026=CARTESIAN_POINT ( 'NONE',  ( -9.166452524254948386, 2.202000163336201410, 48.23896987259320923 ) ) ;
#11034=CARTESIAN_POINT ( 'NONE',  ( -25.32021674380207799, -6.838035406461215437, -48.10016682092218332 ) ) ;
#11037=EDGE_LOOP ( 'NONE', ( #14527, #1368, #8683, #6385, #15079, #2207, #7071, #7114, #5910, #1985 ) ) ;
#11043=DIRECTION ( 'NONE',  ( -0.000000000000000000, 0.000000000000000000, 1.000000000000000000 ) ) ;
#11046=CARTESIAN_POINT ( 'NONE',  ( -25.49999999999998934, -2.249290599286303038, 38.00000000000012079 ) ) ;
#11050=CIRCLE ( 'NONE', #1, 0.5000000000000004441 ) ;
#11053=EDGE_CURVE ( 'NONE', #1708, #4371, #4587, .T. ) ;
#11054=VERTEX_POINT ( 'NONE', #7772 ) ;
#11056=VERTEX_POINT ( 'NONE', #15087 ) ;
#11060=DIRECTION ( 'NONE',  ( 1.000000000000000000, 0.000000000000000000, 0.000000000000000000 ) ) ;
#11066=DIRECTION ( 'NONE',  ( 0.8656763553492639041, 0.5006040828730973224, 0.000000000000000000 ) ) ;
#11068=ORIENTED_EDGE ( 'NONE', *, *, #5650, .T. ) ;
#11075=DIRECTION ( 'NONE',  ( -0.000000000000000000, 1.000000000000000000, 0.000000000000000000 ) ) ;
#11076=TOROIDAL_SURFACE ( 'NONE', #1252, 5.165819364273509073, 0.5000000000000000000 ) ;
#11081=CIRCLE ( 'NONE', #4444, 9.000000000000001776 ) ;
#11084=CARTESIAN_POINT ( 'NONE',  ( -12.14523415828296216, -9.827631355817223024, -48.50000000000012079 ) ) ;
#11085=CARTESIAN_POINT ( 'NONE',  ( -9.444091399599896519, 2.640528280493846580, 48.24517880332174968 ) ) ;
#11090=AXIS2_PLACEMENT_3D ( 'NONE', #2108, #1106, #7038 ) ;
#11091=CARTESIAN_POINT ( 'NONE',  ( -9.037775043065352065, 2.932694901963889489, 58.00000000000012079 ) ) ;
#11096=DIRECTION ( 'NONE',  ( 1.000000000000000000, 0.000000000000000000, 0.000000000000000000 ) ) ;
#11098=ORIENTED_EDGE ( 'NONE', *, *, #12071, .T. ) ;
#11102=EDGE_CURVE ( 'NONE', #8405, #11391, #1393, .T. ) ;
#11104=DIRECTION ( 'NONE',  ( 0.5454721580263448555, -0.8381289428352193260, -0.000000000000000000 ) ) ;
#11106=AXIS2_PLACEMENT_3D ( 'NONE', #6407, #11104, #8475 ) ;
#11107=CARTESIAN_POINT ( 'NONE',  ( -8.958610760419841057, 1.823307968896474840, -58.00000000000012079 ) ) ;
#11109=CARTESIAN_POINT ( 'NONE',  ( -25.27051402993791029, -6.915952606384455414, -48.19241902544784750 ) ) ;
#11111=FACE_OUTER_BOUND ( 'NONE', #1856, .T. ) ;
#11115=DIRECTION ( 'NONE',  ( 0.000000000000000000, 0.000000000000000000, -1.000000000000000000 ) ) ;
#11117=CIRCLE ( 'NONE', #14071, 0.5000000000000004441 ) ;
#11120=LINE ( 'NONE', #1808, #7786 ) ;
#11134=B_SPLINE_CURVE_WITH_KNOTS ( 'NONE', 3,
 ( #3412, #3491, #2334, #10573, #31, #9421, #8269, #9813, #4163, #6201 ),
 .UNSPECIFIED., .F., .F.,
 ( 4, 2, 2, 2, 4 ),
 ( 0.000000000000000000, 0.0003835113287520874100, 0.0007670226575041748200, 0.001150533986256262230, 0.001534045315008349640 ),
 .UNSPECIFIED. ) ;
#11154=ORIENTED_EDGE ( 'NONE', *, *, #11102, .T. ) ;
#11161=EDGE_CURVE ( 'NONE', #5809, #7882, #9009, .T. ) ;
#11165=CARTESIAN_POINT ( 'NONE',  ( -9.041069614211208361, 1.954516911250973932, 47.50000000000011369 ) ) ;
#11169=CARTESIAN_POINT ( 'NONE',  ( -9.354272893020521451, 2.499447352334152050, 47.88483805351501132 ) ) ;
#11182=ORIENTED_EDGE ( 'NONE', *, *, #2930, .T. ) ;
#11184=CARTESIAN_POINT ( 'NONE',  ( -33.07225206673494711, -1.856991049495498425, -48.00000000000012079 ) ) ;
#11187=DIRECTION ( 'NONE',  ( 0.8420378618367723167, 0.5394184268574414576, -0.000000000000000000 ) ) ;
#11195=CARTESIAN_POINT ( 'NONE',  ( -5.290523468902621929, 4.522075770548486418, 48.00000000000012079 ) ) ;
#11201=CARTESIAN_POINT ( 'NONE',  ( -23.19801677984724364, 4.285555568094122414, 47.93908580834070676 ) ) ;
#11206=CARTESIAN_POINT ( 'NONE',  ( -25.99999999999998934, -2.249290599286303927, -47.50000000000012079 ) ) ;
#11209=DIRECTION ( 'NONE',  ( 1.000000000000000000, 0.000000000000000000, 0.000000000000000000 ) ) ;
#11211=VECTOR ( 'NONE', #376, 1000.000000000000000 ) ;
#11224=AXIS2_PLACEMENT_3D ( 'NONE', #12156, #7533, #3769 ) ;
#11230=EDGE_LOOP ( 'NONE', ( #3073, #14609, #3586, #3162 ) ) ;
#11234=VECTOR ( 'NONE', #8247, 1000.000000000000000 ) ;
#11237=ORIENTED_EDGE ( 'NONE', *, *, #4521, .F. ) ;
#11240=EDGE_CURVE ( 'NONE', #10817, #10346, #7239, .T. ) ;
#11242=EDGE_CURVE ( 'NONE', #13978, #10292, #14652, .T. ) ;
#11251=CARTESIAN_POINT ( 'NONE',  ( -24.85140262670387301, -6.666068128078234345, -48.18452149279842445 ) ) ;
#11253=EDGE_CURVE ( 'NONE', #3805, #2373, #10929, .T. ) ;
#11255=ORIENTED_EDGE ( 'NONE', *, *, #6358, .T. ) ;
#11270=CARTESIAN_POINT ( 'NONE',  ( -16.99999999999998579, -2.249290599286303927, -57.50000000000012079 ) ) ;
#11277=VERTEX_POINT ( 'NONE', #7602 ) ;
#11279=EDGE_CURVE ( 'NONE', #13060, #3355, #10734, .T. ) ;
#11281=VERTEX_POINT ( 'NONE', #1605 ) ;
#11284=TOROIDAL_SURFACE ( 'NONE', #7132, 9.500000000000001776, 0.5000000000000000000 ) ;
#11285=DIRECTION ( 'NONE',  ( 0.8656763553493062036, 0.5006040828730242698, 0.000000000000000000 ) ) ;
#11287=CARTESIAN_POINT ( 'NONE',  ( -12.14523415828296216, -9.827631355817223024, -57.50000000000012079 ) ) ;
#11292=VERTEX_POINT ( 'NONE', #8537 ) ;
#11293=CARTESIAN_POINT ( 'NONE',  ( -5.040221427466104132, 4.089237592873841365, 48.50000000000012079 ) ) ;
#11296=CARTESIAN_POINT ( 'NONE',  ( -8.499999999999987566, -2.249290599286303927, -38.50000000000012790 ) ) ;
#11299=CARTESIAN_POINT ( 'NONE',  ( -22.42998452855183444, 4.960558937058127782, -48.26605223428308733 ) ) ;
#11301=EDGE_LOOP ( 'NONE', ( #2826, #11877 ) ) ;
#11302=CARTESIAN_POINT ( 'NONE',  ( -8.787473001628837821, 2.499856724289235554, -48.36782213136056896 ) ) ;
#11312=DIRECTION ( 'NONE',  ( -0.8656763553492640151, -0.5006040828730974335, -0.000000000000000000 ) ) ;
#11317=AXIS2_PLACEMENT_3D ( 'NONE', #7277, #3667, #11966 ) ;
#11323=CIRCLE ( 'NONE', #11090, 0.5000000000000004441 ) ;
#11324=ORIENTED_EDGE ( 'NONE', *, *, #11557, .F. ) ;
#11335=AXIS2_PLACEMENT_3D ( 'NONE', #12937, #6084, #14009 ) ;
#11340=CARTESIAN_POINT ( 'NONE',  ( -8.779641963837230279, 13.70511383897430058, -48.00000000000012079 ) ) ;
#11342=FACE_OUTER_BOUND ( 'NONE', #14472, .T. ) ;
#11353=AXIS2_PLACEMENT_3D ( 'NONE', #11296, #11075, #4293 ) ;
#11356=DIRECTION ( 'NONE',  ( 1.000000000000000000, 0.000000000000000000, 0.000000000000000000 ) ) ;
#11359=LINE ( 'NONE', #10217, #2204 ) ;
#11363=CARTESIAN_POINT ( 'NONE',  ( -9.334567670938534789, -7.621465217813490511, 48.02064173568530236 ) ) ;
#11369=CARTESIAN_POINT ( 'NONE',  ( -1.197457146693678531, -2.220571218158920779, -48.50000000000012079 ) ) ;
#11373=ORIENTED_EDGE ( 'NONE', *, *, #3193, .T. ) ;
#11374=VECTOR ( 'NONE', #1310, 1000.000000000000114 ) ;
#11375=CARTESIAN_POINT ( 'NONE',  ( -16.99999999999998579, -2.249290599286303927, -47.50000000000012079 ) ) ;
#11387=ORIENTED_EDGE ( 'NONE', *, *, #11424, .T. ) ;
#11391=VERTEX_POINT ( 'NONE', #11206 ) ;
#11394=LINE ( 'NONE', #7870, #7809 ) ;
#11396=ORIENTED_EDGE ( 'NONE', *, *, #663, .F. ) ;
#11397=DIRECTION ( 'NONE',  ( 1.000000000000000000, 0.000000000000000000, 0.000000000000000000 ) ) ;
#11400=DIRECTION ( 'NONE',  ( 0.000000000000000000, 0.000000000000000000, -1.000000000000000000 ) ) ;
#11403=EDGE_LOOP ( 'NONE', ( #2069, #968, #6030, #5875 ) ) ;
#11414=DIRECTION ( 'NONE',  ( 0.000000000000000000, -0.000000000000000000, -1.000000000000000000 ) ) ;
#11415=DIRECTION ( 'NONE',  ( 1.000000000000000000, 0.000000000000000000, 0.000000000000000000 ) ) ;
#11418=ORIENTED_EDGE ( 'NONE', *, *, #7268, .T. ) ;
#11424=EDGE_CURVE ( 'NONE', #14061, #9229, #14427, .T. ) ;
#11428=DIRECTION ( 'NONE',  ( 0.8420378618367644341, 0.5394184268574535590, 0.000000000000000000 ) ) ;
#11432=CARTESIAN_POINT ( 'NONE',  ( -3.285520523749251520, 5.681530634151883419, -48.00000000000012079 ) ) ;
#11437=B_SPLINE_CURVE_WITH_KNOTS ( 'NONE', 3,
 ( #5784, #11919, #7086, #11771, #8395, #10549 ),
 .UNSPECIFIED., .F., .F.,
 ( 4, 2, 4 ),
 ( 0.000000000000000000, 0.0003908577252344195446, 0.0007817154504688390891 ),
 .UNSPECIFIED. ) ;
#11443=ORIENTED_EDGE ( 'NONE', *, *, #6370, .T. ) ;
#11449=AXIS2_PLACEMENT_3D ( 'NONE', #10678, #8585, #14372 ) ;
#11451=VERTEX_POINT ( 'NONE', #890 ) ;
#11462=CIRCLE ( 'NONE', #13420, 9.500000000000001776 ) ;
#11463=CARTESIAN_POINT ( 'NONE',  ( -8.982583014919022446, 1.839844381040865562, 48.00000000000012079 ) ) ;
#11467=CYLINDRICAL_SURFACE ( 'NONE', #13185, 0.5000000000000000000 ) ;
#11476=DIRECTION ( 'NONE',  ( 0.5394184268574520047, -0.8420378618367654333, 0.000000000000000000 ) ) ;
#11484=ORIENTED_EDGE ( 'NONE', *, *, #4906, .F. ) ;
#11487=CIRCLE ( 'NONE', #12489, 3.694885682588112896 ) ;
#11493=VECTOR ( 'NONE', #13095, 1000.000000000000000 ) ;
#11494=LINE ( 'NONE', #8122, #3872 ) ;
#11496=FACE_OUTER_BOUND ( 'NONE', #3970, .T. ) ;
#11499=EDGE_CURVE ( 'NONE', #1741, #12265, #7785, .T. ) ;
#11510=CIRCLE ( 'NONE', #11224, 0.5000000000000008882 ) ;
#11517=EDGE_CURVE ( 'NONE', #6801, #3301, #12741, .T. ) ;
#11527=CARTESIAN_POINT ( 'NONE',  ( -23.72465974793126620, 3.743354278179100714, -47.97348817130775700 ) ) ;
#11529=FACE_OUTER_BOUND ( 'NONE', #4492, .T. ) ;
#11537=EDGE_LOOP ( 'NONE', ( #1749, #9642, #9912, #10364 ) ) ;
#11543=DIRECTION ( 'NONE',  ( -0.000000000000000000, -0.000000000000000000, 1.000000000000000000 ) ) ;
#11551=AXIS2_PLACEMENT_3D ( 'NONE', #10925, #7378, #10767 ) ;
#11557=EDGE_CURVE ( 'NONE', #11277, #10236, #14190, .T. ) ;
#11558=ORIENTED_EDGE ( 'NONE', *, *, #13741, .T. ) ;
#11564=FACE_OUTER_BOUND ( 'NONE', #6658, .T. ) ;
#11565=ORIENTED_EDGE ( 'NONE', *, *, #14279, .F. ) ;
#11570=DIRECTION ( 'NONE',  ( -0.5006040828730976555, 0.8656763553492637930, 0.000000000000000000 ) ) ;
#11576=FACE_OUTER_BOUND ( 'NONE', #8526, .T. ) ;
#11579=DIRECTION ( 'NONE',  ( -0.000000000000000000, 0.000000000000000000, 1.000000000000000000 ) ) ;
#11584=CIRCLE ( 'NONE', #3239, 9.000000000000001776 ) ;
#11593=DIRECTION ( 'NONE',  ( 0.000000000000000000, 0.000000000000000000, 1.000000000000000000 ) ) ;
#11597=CARTESIAN_POINT ( 'NONE',  ( -3.190546569013415379, 0.8906624217387615339, -57.50000000000012079 ) ) ;
#11599=DIRECTION ( 'NONE',  ( 1.000000000000000000, 0.000000000000000000, 0.000000000000000000 ) ) ;
#11607=ORIENTED_EDGE ( 'NONE', *, *, #7012, .T. ) ;
#11616=FACE_OUTER_BOUND ( 'NONE', #10784, .T. ) ;
#11619=DIRECTION ( 'NONE',  ( 1.000000000000000000, 0.000000000000000000, 0.000000000000000000 ) ) ;
#11625=CARTESIAN_POINT ( 'NONE',  ( -9.037775043065350289, 2.932694901963889933, 48.50000000000012079 ) ) ;
#11640=AXIS2_PLACEMENT_3D ( 'NONE', #670, #10149, #14606 ) ;
#11641=PLANE ( 'NONE',  #10029 ) ;
#11650=EDGE_LOOP ( 'NONE', ( #2496, #13568, #8337, #11154, #5188 ) ) ;
#11674=ORIENTED_EDGE ( 'NONE', *, *, #12243, .F. ) ;
#11693=TOROIDAL_SURFACE ( 'NONE', #15139, 5.165819364273509073, 0.5000000000000000000 ) ;
#11708=CARTESIAN_POINT ( 'NONE',  ( -10.96079405803985729, -9.021238043844263643, -48.26696389624903816 ) ) ;
#11713=FACE_OUTER_BOUND ( 'NONE', #14083, .T. ) ;
#11715=DIRECTION ( 'NONE',  ( 0.5006040828730242698, -0.8656763553493062036, 0.000000000000000000 ) ) ;
#11720=VERTEX_POINT ( 'NONE', #5112 ) ;
#11721=DIRECTION ( 'NONE',  ( 1.000000000000000000, 0.000000000000000000, 0.000000000000000000 ) ) ;
#11722=CIRCLE ( 'NONE', #6078, 0.5000000000000004441 ) ;
#11723=VERTEX_POINT ( 'NONE', #4165 ) ;
#11728=CARTESIAN_POINT ( 'NONE',  ( -8.842479278987921631, -7.118053859731281463, 48.00000000000012079 ) ) ;
#11729=LINE ( 'NONE', #2648, #10006 ) ;
#11734=CYLINDRICAL_SURFACE ( 'NONE', #14698, 4.665819364273509073 ) ;
#11742=VECTOR ( 'NONE', #6028, 1000.000000000000000 ) ;
#11752=ADVANCED_FACE ( 'NONE', ( #14635 ), #3090, .T. ) ;
#11753=AXIS2_PLACEMENT_3D ( 'NONE', #4419, #8964, #6887 ) ;
#11756=DIRECTION ( 'NONE',  ( -0.5394184268574385710, 0.8420378618367740930, 0.000000000000000000 ) ) ;
#11766=EDGE_CURVE ( 'NONE', #10853, #15152, #8865, .T. ) ;
#11768=CARTESIAN_POINT ( 'NONE',  ( -24.72817752516938228, 2.363221963240404566, -47.50000000000012079 ) ) ;
#11771=CARTESIAN_POINT ( 'NONE',  ( -8.655068852960594583, 2.300722221922764543, 48.05421924268924272 ) ) ;
#11773=ADVANCED_FACE ( 'NONE', ( #3407 ), #11693, .T. ) ;
#11775=CARTESIAN_POINT ( 'NONE',  ( -9.456839514482961562, 2.659958822950721835, -48.50000000000012079 ) ) ;
#11776=CARTESIAN_POINT ( 'NONE',  ( -24.96222495693456978, -7.431276100536581275, -58.00000000000012079 ) ) ;
#11783=ORIENTED_EDGE ( 'NONE', *, *, #12051, .T. ) ;
#11788=DIRECTION ( 'NONE',  ( -0.000000000000000000, -0.000000000000000000, 1.000000000000000000 ) ) ;
#11793=CARTESIAN_POINT ( 'NONE',  ( 0.6601805061683232445, -1.030548743169294346, -57.50000000000012079 ) ) ;
#11797=CARTESIAN_POINT ( 'NONE',  ( -25.01741698508091005, -6.338425579613558014, -47.50000000000012079 ) ) ;
#11808=CARTESIAN_POINT ( 'NONE',  ( -24.54316048551696028, -7.158540021523408292, 48.50000000000011369 ) ) ;
#11826=CYLINDRICAL_SURFACE ( 'NONE', #3029, 4.665819364273509073 ) ;
#11828=DIRECTION ( 'NONE',  ( 0.000000000000000000, 0.000000000000000000, 1.000000000000000000 ) ) ;
#11835=DIRECTION ( 'NONE',  ( -0.5394184268574404584, 0.8420378618367728718, 0.000000000000000000 ) ) ;
#11839=EDGE_CURVE ( 'NONE', #8112, #1741, #12185, .T. ) ;
#11844=AXIS2_PLACEMENT_3D ( 'NONE', #6667, #2130, #11356 ) ;
#11854=AXIS2_PLACEMENT_3D ( 'NONE', #752, #13616, #7771 ) ;
#11855=CARTESIAN_POINT ( 'NONE',  ( -24.72817752516938228, 2.363221963240404566, 47.50000000000012079 ) ) ;
#11866=CARTESIAN_POINT ( 'NONE',  ( -16.99999999999998579, -2.249290599286303927, -58.00000000000012079 ) ) ;
#11869=CIRCLE ( 'NONE', #12121, 9.000000000000001776 ) ;
#11877=ORIENTED_EDGE ( 'NONE', *, *, #5650, .F. ) ;
#11887=TOROIDAL_SURFACE ( 'NONE', #4006, 3.694885682588112452, 0.5000000000000000000 ) ;
#11895=EDGE_CURVE ( 'NONE', #15152, #11056, #7271, .T. ) ;
#11900=CARTESIAN_POINT ( 'NONE',  ( -16.99999999999998579, -2.249290599286303927, -50.00000000000012079 ) ) ;
#11901=DIRECTION ( 'NONE',  ( 1.224646799147353207E-16, -1.000000000000000000, 0.000000000000000000 ) ) ;
#11905=ORIENTED_EDGE ( 'NONE', *, *, #8900, .F. ) ;
#11912=ORIENTED_EDGE ( 'NONE', *, *, #12527, .F. ) ;
#11915=CARTESIAN_POINT ( 'NONE',  ( -21.85476584171713199, 5.329050157244537900, -48.50000000000012079 ) ) ;
#11919=CARTESIAN_POINT ( 'NONE',  ( -8.787473001628837821, 2.499856724289235554, 48.36782213136056896 ) ) ;
#11923=CARTESIAN_POINT ( 'NONE',  ( -8.537170960192302260, 2.067018546614596719, -47.50000000000012079 ) ) ;
#11924=ORIENTED_EDGE ( 'NONE', *, *, #6171, .F. ) ;
#11925=ADVANCED_FACE ( 'NONE', ( #859 ), #6751, .F. ) ;
#11935=CARTESIAN_POINT ( 'NONE',  ( -10.31821280924931372, -8.288623256088383684, -47.74919337097148286 ) ) ;
#11936=CARTESIAN_POINT ( 'NONE',  ( -24.96222495693456978, -7.431276100536581275, 48.50000000000012079 ) ) ;
#11937=DIRECTION ( 'NONE',  ( -0.000000000000000000, -0.000000000000000000, 1.000000000000000000 ) ) ;
#11940=DIRECTION ( 'NONE',  ( -0.000000000000000000, 0.000000000000000000, 1.000000000000000000 ) ) ;
#11946=DIRECTION ( 'NONE',  ( 0.000000000000000000, 0.000000000000000000, -1.000000000000000000 ) ) ;
#11947=ORIENTED_EDGE ( 'NONE', *, *, #13889, .F. ) ;
#11949=FACE_OUTER_BOUND ( 'NONE', #10972, .T. ) ;
#11966=DIRECTION ( 'NONE',  ( 1.000000000000000000, 0.000000000000000000, 0.000000000000000000 ) ) ;
#11976=ADVANCED_FACE ( 'NONE', ( #1172 ), #14259, .T. ) ;
#11979=CARTESIAN_POINT ( 'NONE',  ( -16.99999999999998579, -2.249290599286303927, -58.00000000000012079 ) ) ;
#11987=CARTESIAN_POINT ( 'NONE',  ( -3.035218482312739496, 5.248692456477230373, -57.50000000000012079 ) ) ;
#11993=PLANE ( 'NONE',  #6425 ) ;
#11997=EDGE_CURVE ( 'NONE', #9911, #5507, #4058, .T. ) ;
#12005=EDGE_LOOP ( 'NONE', ( #13683, #11255 ) ) ;
#12008=VERTEX_POINT ( 'NONE', #3560 ) ;
#12015=AXIS2_PLACEMENT_3D ( 'NONE', #9475, #160, #4850 ) ;
#12019=CARTESIAN_POINT ( 'NONE',  ( -24.55590860040002710, -7.139109479066534369, 48.24517880332174968 ) ) ;
#12031=TOROIDAL_SURFACE ( 'NONE', #8593, 3.694885682587998765, 0.5000000000000000000 ) ;
#12032=AXIS2_PLACEMENT_3D ( 'NONE', #9500, #11946, #11721 ) ;
#12033=B_SPLINE_CURVE_WITH_KNOTS ( 'NONE', 3,
 ( #2961, #4101, #493, #1507, #14438, #356 ),
 .UNSPECIFIED., .F., .F.,
 ( 4, 2, 4 ),
 ( 0.000000000000000000, 0.0003908577252344191651, 0.0007817154504688383302 ),
 .UNSPECIFIED. ) ;
#12037=CARTESIAN_POINT ( 'NONE',  ( -16.99999999999998579, -2.249290599286303927, -47.50000000000012079 ) ) ;
#12039=EDGE_CURVE ( 'NONE', #7398, #2221, #6051, .T. ) ;
#12047=ORIENTED_EDGE ( 'NONE', *, *, #9149, .T. ) ;
#12048=CARTESIAN_POINT ( 'NONE',  ( -11.83418063572647760, -2.249290599286303927, 58.00000000000012079 ) ) ;
#12049=VERTEX_POINT ( 'NONE', #14482 ) ;
#12051=EDGE_CURVE ( 'NONE', #13513, #7624, #13541, .T. ) ;
#12054=CARTESIAN_POINT ( 'NONE',  ( -30.80945343098651890, -5.389243620311580329, 58.00000000000012079 ) ) ;
#12061=ORIENTED_EDGE ( 'NONE', *, *, #165, .F. ) ;
#12066=( BOUNDED_SURFACE ( )  B_SPLINE_SURFACE ( 3, 2, ( 
 ( #10965, #3447, #3530 ),
 ( #415, #5115, #14503 ),
 ( #7648, #5414, #705 ),
 ( #1798, #7800, #2956 ),
 ( #11109, #11251, #5499 ),
 ( #11034, #1939, #12342 ),
 ( #4249, #2870, #13407 ),
 ( #12493, #5336, #6636 ),
 ( #10033, #14795, #10187 ),
 ( #4020, #4322, #6490 ) ),
 .UNSPECIFIED., .F., .F., .F. ) 
 B_SPLINE_SURFACE_WITH_KNOTS ( ( 4, 2, 2, 2, 4 ),
 ( 3, 3 ),
 ( 0.0006711510808134562266, 0.001062132081067026709, 0.001453113081320597409, 0.001844094081574168108, 0.002235075081827738591 ),
 ( 0.000000000000000000, 1.000000000000000000 ),
 .UNSPECIFIED. ) 
 GEOMETRIC_REPRESENTATION_ITEM ( )  RATIONAL_B_SPLINE_SURFACE ( (
 ( 1.000000000000000000, 0.7254762501099963901, 1.000000000000000000),
 ( 1.000000000000000000, 0.7255094664176422459, 1.000000000000000000),
 ( 1.000000000000000000, 0.7239949553644952074, 1.000000000000000000),
 ( 1.000000000000000000, 0.7190573720639429345, 1.000000000000000000),
 ( 1.000000000000000000, 0.7156412189950915881, 1.000000000000000000),
 ( 1.000000000000000000, 0.7094102539594338008, 1.000000000000000000),
 ( 1.000000000000000000, 0.7066203625162998936, 1.000000000000000000),
 ( 1.000000000000000000, 0.7042417591947802702, 1.000000000000000000),
 ( 1.000000000000000000, 0.7046402682201203804, 1.000000000000000000),
 ( 1.000000000000000000, 0.7071067811865500152, 1.000000000000000000) ) ) 
 REPRESENTATION_ITEM ( '' )  SURFACE ( )  );
#12067=CARTESIAN_POINT ( 'NONE',  ( -22.54958699671023581, 4.838095916862976686, 48.21133583021728697 ) ) ;
#12070=AXIS2_PLACEMENT_3D ( 'NONE', #2274, #4341, #11415 ) ;
#12071=EDGE_CURVE ( 'NONE', #9229, #1375, #4649, .T. ) ;
#12074=CARTESIAN_POINT ( 'NONE',  ( -11.86108202630535224, -9.639858853941328576, 48.38337049880509255 ) ) ;
#12075=ORIENTED_EDGE ( 'NONE', *, *, #8610, .F. ) ;
#12080=CIRCLE ( 'NONE', #5692, 0.5000000000000004441 ) ;
#12082=CYLINDRICAL_SURFACE ( 'NONE', #3715, 0.5000000000000004441 ) ;
#12085=LINE ( 'NONE', #1468, #11493 ) ;
#12092=CARTESIAN_POINT ( 'NONE',  ( -3.190546569013415379, 0.8906624217387615339, -48.00000000000012079 ) ) ;
#12094=AXIS2_PLACEMENT_3D ( 'NONE', #7195, #4889, #9592 ) ;
#12098=CARTESIAN_POINT ( 'NONE',  ( -11.05444845021228595, -9.014367880605227867, -48.04486892757390848 ) ) ;
#12101=TOROIDAL_SURFACE ( 'NONE', #3237, 8.500000000000000000, 0.5000000000000000000 ) ;
#12103=AXIS2_PLACEMENT_3D ( 'NONE', #11293, #9159, #748 ) ;
#12114=DIRECTION ( 'NONE',  ( 1.000000000000000000, 0.000000000000000000, 0.000000000000000000 ) ) ;
#12121=AXIS2_PLACEMENT_3D ( 'NONE', #10302, #7611, #6453 ) ;
#12124=CIRCLE ( 'NONE', #12620, 0.5000000000000003331 ) ;
#12125=ORIENTED_EDGE ( 'NONE', *, *, #11499, .F. ) ;
#12136=EDGE_CURVE ( 'NONE', #6074, #9111, #12425, .T. ) ;
#12144=ORIENTED_EDGE ( 'NONE', *, *, #12527, .T. ) ;
#12150=DIRECTION ( 'NONE',  ( 0.000000000000000000, -0.000000000000000000, -1.000000000000000000 ) ) ;
#12155=VERTEX_POINT ( 'NONE', #10394 ) ;
#12156=CARTESIAN_POINT ( 'NONE',  ( -28.95977857253363297, -8.587818791446675704, 48.50000000000012079 ) ) ;
#12157=DIRECTION ( 'NONE',  ( -0.000000000000000000, -0.000000000000000000, 1.000000000000000000 ) ) ;
#12161=VERTEX_POINT ( 'NONE', #12465 ) ;
#12162=ORIENTED_EDGE ( 'NONE', *, *, #8304, .T. ) ;
#12163=DIRECTION ( 'NONE',  ( 0.000000000000000000, 0.000000000000000000, -1.000000000000000000 ) ) ;
#12178=CARTESIAN_POINT ( 'NONE',  ( 0.9298897195970434737, -1.451567674087680837, 48.50000000000012079 ) ) ;
#12179=DIRECTION ( 'NONE',  ( 1.000000000000000000, 0.000000000000000000, 0.000000000000000000 ) ) ;
#12183=EDGE_CURVE ( 'NONE', #11054, #4463, #13657, .T. ) ;
#12185=CIRCLE ( 'NONE', #1626, 3.694885682587998765 ) ;
#12189=CARTESIAN_POINT ( 'NONE',  ( -21.16581936427349575, -2.249290599286303483, 50.00000000000012079 ) ) ;
#12193=CARTESIAN_POINT ( 'NONE',  ( -16.99999999999998579, -2.249290599286303927, 48.00000000000012079 ) ) ;
#12205=ORIENTED_EDGE ( 'NONE', *, *, #13830, .T. ) ;
#12211=CYLINDRICAL_SURFACE ( 'NONE', #10822, 0.5000000000000000000 ) ;
#12217=CARTESIAN_POINT ( 'NONE',  ( -25.46282903980766932, -6.565599745187317815, 57.50000000000012079 ) ) ;
#12243=EDGE_CURVE ( 'NONE', #1375, #9911, #4538, .T. ) ;
#12253=ADVANCED_FACE ( 'NONE', ( #11616 ), #769, .T. ) ;
#12265=VERTEX_POINT ( 'NONE', #6691 ) ;
#12267=ORIENTED_EDGE ( 'NONE', *, *, #2430, .F. ) ;
#12274=EDGE_CURVE ( 'NONE', #7187, #8918, #11584, .T. ) ;
#12280=CARTESIAN_POINT ( 'NONE',  ( -24.90998783373886738, 2.881753107372537759, -48.00000000000012079 ) ) ;
#12284=ORIENTED_EDGE ( 'NONE', *, *, #3452, .F. ) ;
#12288=EDGE_CURVE ( 'NONE', #7044, #3003, #522, .T. ) ;
#12294=DIRECTION ( 'NONE',  ( 0.8656763553492640151, 0.5006040828730974335, 0.000000000000000000 ) ) ;
#12296=AXIS2_PLACEMENT_3D ( 'NONE', #693, #10325, #7866 ) ;
#12305=CARTESIAN_POINT ( 'NONE',  ( -12.14523415828296216, -9.827631355817223024, -48.00000000000012079 ) ) ;
#12310=AXIS2_PLACEMENT_3D ( 'NONE', #8132, #3736, #15211 ) ;
#12312=EDGE_CURVE ( 'NONE', #3688, #9584, #10850, .T. ) ;
#12315=CIRCLE ( 'NONE', #14771, 4.194885682588113340 ) ;
#12317=ORIENTED_EDGE ( 'NONE', *, *, #13641, .F. ) ;
#12330=ORIENTED_EDGE ( 'NONE', *, *, #8518, .F. ) ;
#12332=CARTESIAN_POINT ( 'NONE',  ( -12.41494337171168283, -9.406612424898836977, 58.00000000000012079 ) ) ;
#12334=DIRECTION ( 'NONE',  ( 1.000000000000000000, 0.000000000000000000, 0.000000000000000000 ) ) ;
#12337=ADVANCED_FACE ( 'NONE', ( #4846, #4692 ), #9395, .F. ) ;
#12341=FACE_OUTER_BOUND ( 'NONE', #5779, .T. ) ;
#12342=CARTESIAN_POINT ( 'NONE',  ( -24.73660316015754290, -6.848489080522048411, -47.70033363922482295 ) ) ;
#12345=TOROIDAL_SURFACE ( 'NONE', #3215, 1.000000000000000000, 0.5000000000000000000 ) ;
#12351=FACE_OUTER_BOUND ( 'NONE', #7167, .T. ) ;
#12375=DIRECTION ( 'NONE',  ( 0.000000000000000000, 0.000000000000000000, -1.000000000000000000 ) ) ;
#12386=ORIENTED_EDGE ( 'NONE', *, *, #7582, .F. ) ;
#12391=CARTESIAN_POINT ( 'NONE',  ( -16.99999999999998579, -2.249290599286303927, -38.00000000000012079 ) ) ;
#12401=DIRECTION ( 'NONE',  ( 0.8656763553493062036, 0.5006040828730242698, 0.000000000000000000 ) ) ;
#12403=DIRECTION ( 'NONE',  ( 1.000000000000000000, 0.000000000000000000, 0.000000000000000000 ) ) ;
#12405=DIRECTION ( 'NONE',  ( -0.000000000000000000, 0.000000000000000000, 1.000000000000000000 ) ) ;
#12408=ADVANCED_FACE ( 'NONE', ( #1228 ), #11993, .F. ) ;
#12414=ORIENTED_EDGE ( 'NONE', *, *, #1328, .T. ) ;
#12419=ORIENTED_EDGE ( 'NONE', *, *, #4469, .T. ) ;
#12421=DIRECTION ( 'NONE',  ( -0.8420378618367728718, -0.5394184268574404584, 0.000000000000000000 ) ) ;
#12425=CIRCLE ( 'NONE', #5810, 8.500000000000000000 ) ;
#12432=ORIENTED_EDGE ( 'NONE', *, *, #2468, .F. ) ;
#12450=ORIENTED_EDGE ( 'NONE', *, *, #10388, .T. ) ;
#12457=ORIENTED_EDGE ( 'NONE', *, *, #12757, .F. ) ;
#12460=DIRECTION ( 'NONE',  ( 1.000000000000000000, 0.000000000000000000, 0.000000000000000000 ) ) ;
#12462=ADVANCED_FACE ( 'NONE', ( #14676 ), #10932, .T. ) ;
#12463=EDGE_CURVE ( 'NONE', #10969, #13205, #4130, .T. ) ;
#12465=CARTESIAN_POINT ( 'NONE',  ( -32.80254285330622821, -2.278009980413885582, 58.00000000000012079 ) ) ;
#12467=AXIS2_PLACEMENT_3D ( 'NONE', #1957, #6654, #805 ) ;
#12472=FACE_OUTER_BOUND ( 'NONE', #11037, .T. ) ;
#12477=DIRECTION ( 'NONE',  ( 0.000000000000000000, 0.000000000000000000, 1.000000000000000000 ) ) ;
#12478=EDGE_LOOP ( 'NONE', ( #6365, #9168, #5574, #12802 ) ) ;
#12482=ADVANCED_FACE ( 'NONE', ( #13524 ), #6206, .T. ) ;
#12487=EDGE_LOOP ( 'NONE', ( #1943, #2678, #1740, #10602 ) ) ;
#12489=AXIS2_PLACEMENT_3D ( 'NONE', #2196, #11414, #10354 ) ;
#12493=CARTESIAN_POINT ( 'NONE',  ( -25.40673215887140657, -6.684475985750503391, -48.01308457333527002 ) ) ;
#12496=ORIENTED_EDGE ( 'NONE', *, *, #1335, .F. ) ;
#12506=DIRECTION ( 'NONE',  ( 1.000000000000000000, 0.000000000000000000, 0.000000000000000000 ) ) ;
#12508=ADVANCED_FACE ( 'NONE', ( #13832, #12525 ), #1970, .T. ) ;
#12513=ORIENTED_EDGE ( 'NONE', *, *, #6666, .T. ) ;
#12514=CIRCLE ( 'NONE', #4902, 0.5000000000000004441 ) ;
#12519=CARTESIAN_POINT ( 'NONE',  ( 1.004339113574583608, 0.8906624217387615339, -57.50000000000012079 ) ) ;
#12520=ADVANCED_FACE ( 'NONE', ( #3063 ), #4278, .F. ) ;
#12521=CARTESIAN_POINT ( 'NONE',  ( -9.456839514482961562, 2.659958822950722723, 58.00000000000012079 ) ) ;
#12525=FACE_OUTER_BOUND ( 'NONE', #10531, .T. ) ;
#12527=EDGE_CURVE ( 'NONE', #12265, #6058, #5703, .T. ) ;
#12532=CARTESIAN_POINT ( 'NONE',  ( -7.499999999999985789, -2.249290599286303927, 48.00000000000012079 ) ) ;
#12538=FACE_OUTER_BOUND ( 'NONE', #11230, .T. ) ;
#12546=CARTESIAN_POINT ( 'NONE',  ( -1.197457146693716057, -2.220571218158943427, -48.00000000000012079 ) ) ;
#12557=EDGE_LOOP ( 'NONE', ( #4277, #9397, #9980, #13158 ) ) ;
#12565=AXIS2_PLACEMENT_3D ( 'NONE', #4025, #8799, #13495 ) ;
#12567=DIRECTION ( 'NONE',  ( 1.000000000000000000, 0.000000000000000000, 0.000000000000000000 ) ) ;
#12568=LINE ( 'NONE', #4089, #5420 ) ;
#12571=EDGE_CURVE ( 'NONE', #5507, #5398, #1753, .T. ) ;
#12598=DIRECTION ( 'NONE',  ( 1.000000000000000000, 0.000000000000000000, 0.000000000000000000 ) ) ;
#12604=CARTESIAN_POINT ( 'NONE',  ( -12.14523415828296216, -9.827631355817223024, 48.50000000000012079 ) ) ;
#12608=EDGE_CURVE ( 'NONE', #10969, #490, #3726, .T. ) ;
#12609=PLANE ( 'NONE',  #2940 ) ;
#12616=DIRECTION ( 'NONE',  ( -0.8586863916854874379, 0.5125013958363018318, 0.000000000000000000 ) ) ;
#12620=AXIS2_PLACEMENT_3D ( 'NONE', #11923, #1388, #9638 ) ;
#12626=DIRECTION ( 'NONE',  ( 0.000000000000000000, 0.000000000000000000, -1.000000000000000000 ) ) ;
#12632=CIRCLE ( 'NONE', #14076, 5.165819364273509073 ) ;
#12635=CARTESIAN_POINT ( 'NONE',  ( -8.982583014919022446, 1.839844381040865562, 47.50000000000012079 ) ) ;
#12643=CARTESIAN_POINT ( 'NONE',  ( -16.99999999999998579, -2.249290599286303927, -57.50000000000012079 ) ) ;
#12645=DIRECTION ( 'NONE',  ( 0.000000000000000000, -0.000000000000000000, -1.000000000000000000 ) ) ;
#12650=CARTESIAN_POINT ( 'NONE',  ( -25.46282903980766932, -6.565599745187317815, 58.00000000000012079 ) ) ;
#12655=DIRECTION ( 'NONE',  ( 1.000000000000000000, 0.000000000000000000, 0.000000000000000000 ) ) ;
#12661=DIRECTION ( 'NONE',  ( 0.5394184268574535590, -0.8420378618367644341, 0.000000000000000000 ) ) ;
#12667=ORIENTED_EDGE ( 'NONE', *, *, #2058, .T. ) ;
#12670=DIRECTION ( 'NONE',  ( 0.000000000000000000, -0.000000000000000000, -1.000000000000000000 ) ) ;
#12671=ORIENTED_EDGE ( 'NONE', *, *, #15218, .F. ) ;
#12673=DIRECTION ( 'NONE',  ( -0.8656763553493057595, -0.5006040828730249359, 0.000000000000000000 ) ) ;
#12674=B_SPLINE_CURVE_WITH_KNOTS ( 'NONE', 3,
 ( #1484, #13114, #8421, #13182, #2569, #7256, #2637, #12019, #10879, #13393 ),
 .UNSPECIFIED., .F., .F.,
 ( 4, 2, 2, 2, 4 ),
 ( 0.000000000000000000, 0.0003835113287520874100, 0.0007670226575041748200, 0.001150533986256262230, 0.001534045315008349640 ),
 .UNSPECIFIED. ) ;
#12685=CARTESIAN_POINT ( 'NONE',  ( -10.04144563215826835, -7.967033079555101871, 47.93156476714629122 ) ) ;
#12688=FACE_OUTER_BOUND ( 'NONE', #5153, .T. ) ;
#12693=CARTESIAN_POINT ( 'NONE',  ( -25.15752072101216896, 2.619472661158628313, -48.00000000000012079 ) ) ;
#12699=EDGE_CURVE ( 'NONE', #8918, #7187, #14545, .T. ) ;
#12700=ORIENTED_EDGE ( 'NONE', *, *, #7723, .F. ) ;
#12703=PLANE ( 'NONE',  #14488 ) ;
#12708=EDGE_CURVE ( 'NONE', #864, #11054, #5716, .T. ) ;
#12713=CARTESIAN_POINT ( 'NONE',  ( -3.190546569013415379, 0.8906624217387615339, 48.00000000000012079 ) ) ;
#12714=EDGE_LOOP ( 'NONE', ( #434, #2765, #8409, #5893 ) ) ;
#12719=CARTESIAN_POINT ( 'NONE',  ( -9.456985518117400957, -7.172040337370347629, -47.50000001881890910 ) ) ;
#12722=VECTOR ( 'NONE', #13224, 1000.000000000000000 ) ;
#12740=AXIS2_PLACEMENT_3D ( 'NONE', #9419, #14110, #3562 ) ;
#12741=CIRCLE ( 'NONE', #6804, 0.4999999999999999445 ) ;
#12753=CARTESIAN_POINT ( 'NONE',  ( -25.40901433244242114, -6.686340856221296036, -48.00000000000012079 ) ) ;
#12756=CARTESIAN_POINT ( 'NONE',  ( -12.83418063572647760, -2.249290599286303927, 50.50000000000012079 ) ) ;
#12757=EDGE_CURVE ( 'NONE', #1708, #4049, #1805, .T. ) ;
#12760=CARTESIAN_POINT ( 'NONE',  ( -28.70947653109703168, -9.020656969121420232, 48.50000000000012079 ) ) ;
#12769=CARTESIAN_POINT ( 'NONE',  ( -8.842479278987875446, -7.118053859731355182, 48.00000000000012079 ) ) ;
#12770=AXIS2_PLACEMENT_3D ( 'NONE', #14112, #11715, #8192 ) ;
#12775=CARTESIAN_POINT ( 'NONE',  ( -25.46282903980766932, -6.565599745187317815, -57.50000000000012079 ) ) ;
#12776=VERTEX_POINT ( 'NONE', #5744 ) ;
#12782=EDGE_LOOP ( 'NONE', ( #12432, #5698, #10723, #13620 ) ) ;
#12787=ORIENTED_EDGE ( 'NONE', *, *, #7582, .T. ) ;
#12792=VERTEX_POINT ( 'NONE', #2187 ) ;
#12796=ORIENTED_EDGE ( 'NONE', *, *, #11895, .T. ) ;
#12798=CARTESIAN_POINT ( 'NONE',  ( -8.787473001628837821, 2.499856724289235554, 48.50000000000012079 ) ) ;
#12800=CARTESIAN_POINT ( 'NONE',  ( -10.04144563215826835, -7.967033079554944663, -47.93156476714629122 ) ) ;
#12801=CARTESIAN_POINT ( 'NONE',  ( -11.83418063572647760, -2.249290599286303927, 57.50000000000012079 ) ) ;
#12802=ORIENTED_EDGE ( 'NONE', *, *, #2587, .F. ) ;
#12805=CIRCLE ( 'NONE', #4177, 4.194885682587998765 ) ;
#12806=DIRECTION ( 'NONE',  ( -0.5394184268574404584, 0.8420378618367728718, 0.000000000000000000 ) ) ;
#12811=EDGE_LOOP ( 'NONE', ( #8114, #8274, #7224, #3609 ) ) ;
#12812=AXIS2_PLACEMENT_3D ( 'NONE', #13606, #6519, #5375 ) ;
#12813=DIRECTION ( 'NONE',  ( 0.000000000000000000, 0.000000000000000000, -1.000000000000000000 ) ) ;
#12817=ORIENTED_EDGE ( 'NONE', *, *, #8948, .T. ) ;
#12819=FACE_OUTER_BOUND ( 'NONE', #14875, .T. ) ;
#12820=ADVANCED_FACE ( 'NONE', ( #11564 ), #2102, .T. ) ;
#12822=AXIS2_PLACEMENT_3D ( 'NONE', #3222, #7925, #12616 ) ;
#12825=PLANE ( 'NONE',  #1174 ) ;
#12827=CARTESIAN_POINT ( 'NONE',  ( -16.99999999999998579, -2.249290599286303927, 47.50000000000012079 ) ) ;
#12829=CARTESIAN_POINT ( 'NONE',  ( -21.85476584171713199, 5.329050157244537900, -48.50000000000012079 ) ) ;
#12849=DIRECTION ( 'NONE',  ( 1.000000000000000000, 0.000000000000000000, 0.000000000000000000 ) ) ;
#12853=LINE ( 'NONE', #6991, #1069 ) ;
#12858=ORIENTED_EDGE ( 'NONE', *, *, #4052, .F. ) ;
#12859=CIRCLE ( 'NONE', #14798, 3.694885682587998765 ) ;
#12871=CARTESIAN_POINT ( 'NONE',  ( -7.999999999999986677, -2.249290599286305259, -38.50000000000012790 ) ) ;
#12879=VERTEX_POINT ( 'NONE', #3183 ) ;
#12895=ORIENTED_EDGE ( 'NONE', *, *, #6036, .F. ) ;
#12906=CARTESIAN_POINT ( 'NONE',  ( -24.60804510916187837, -7.057608296800744085, 47.99579695943414492 ) ) ;
#12916=ORIENTED_EDGE ( 'NONE', *, *, #663, .T. ) ;
#12924=DIRECTION ( 'NONE',  ( 0.8420378618367735379, 0.5394184268574396812, 9.357418084440779321E-16 ) ) ;
#12925=CARTESIAN_POINT ( 'NONE',  ( -3.190546569013415379, 0.8906624217387615339, 48.00000000000012079 ) ) ;
#12931=ORIENTED_EDGE ( 'NONE', *, *, #5395, .F. ) ;
#12937=CARTESIAN_POINT ( 'NONE',  ( 0.000000000000000000, 0.000000000000000000, 38.00000000000012079 ) ) ;
#12944=FACE_OUTER_BOUND ( 'NONE', #10541, .T. ) ;
#12959=FACE_OUTER_BOUND ( 'NONE', #13755, .T. ) ;
#12961=CARTESIAN_POINT ( 'NONE',  ( -16.99999999999998579, -2.249290599286303927, 47.50000000000012079 ) ) ;
#12963=ORIENTED_EDGE ( 'NONE', *, *, #349, .F. ) ;
#12978=DIRECTION ( 'NONE',  ( -0.000000000000000000, -0.000000000000000000, 1.000000000000000000 ) ) ;
#12979=CARTESIAN_POINT ( 'NONE',  ( -25.40673215887140657, -6.684475985750503391, 48.01308457333527002 ) ) ;
#12985=ORIENTED_EDGE ( 'NONE', *, *, #8967, .T. ) ;
#12990=ORIENTED_EDGE ( 'NONE', *, *, #5484, .F. ) ;
#12992=ADVANCED_FACE ( 'NONE', ( #11949 ), #13084, .T. ) ;
#13005=CARTESIAN_POINT ( 'NONE',  ( -30.80945343098651890, -5.389243620311580329, -57.50000000000012079 ) ) ;
#13006=EDGE_LOOP ( 'NONE', ( #9950, #2584, #10835, #6758 ) ) ;
#13010=DIRECTION ( 'NONE',  ( -0.000000000000000000, -0.000000000000000000, 1.000000000000000000 ) ) ;
#13018=CARTESIAN_POINT ( 'NONE',  ( -25.99999999999998934, -2.249290599286303927, -58.00000000000012079 ) ) ;
#13029=CARTESIAN_POINT ( 'NONE',  ( -1.197457146693678531, -2.220571218158920779, 48.00000000000012079 ) ) ;
#13032=DIRECTION ( 'NONE',  ( 1.000000000000000000, 0.000000000000000000, 0.000000000000000000 ) ) ;
#13033=DIRECTION ( 'NONE',  ( -0.000000000000000000, 1.000000000000000000, 0.000000000000000000 ) ) ;
#13051=CARTESIAN_POINT ( 'NONE',  ( -24.80190065418678458, -6.760980545838084943, 48.43121057161747700 ) ) ;
#13052=AXIS2_PLACEMENT_3D ( 'NONE', #3879, #13343, #9820 ) ;
#13056=UNCERTAINTY_MEASURE_WITH_UNIT (LENGTH_MEASURE( 1.000000000000000082E-05 ), #10177, 'distance_accuracy_value', 'NONE');
#13059=ORIENTED_EDGE ( 'NONE', *, *, #3292, .F. ) ;
#13060=VERTEX_POINT ( 'NONE', #15151 ) ;
#13075=ORIENTED_EDGE ( 'NONE', *, *, #4673, .T. ) ;
#13077=EDGE_LOOP ( 'NONE', ( #8477, #14333, #6304, #546 ) ) ;
#13079=VERTEX_POINT ( 'NONE', #4447 ) ;
#13084=TOROIDAL_SURFACE ( 'NONE', #4972, 3.694885682587998765, 0.5000000000000000000 ) ;
#13088=DIRECTION ( 'NONE',  ( 0.8420378618367728718, 0.5394184268574404584, 0.000000000000000000 ) ) ;
#13095=DIRECTION ( 'NONE',  ( 0.000000000000000000, 0.000000000000000000, -1.000000000000000000 ) ) ;
#13099=EDGE_CURVE ( 'NONE', #13646, #3062, #10130, .T. ) ;
#13100=EDGE_LOOP ( 'NONE', ( #8010, #5834, #14677, #12267 ) ) ;
#13104=CARTESIAN_POINT ( 'NONE',  ( -11.04362772831848716, -9.031687326780717839, -48.03392779025379156 ) ) ;
#13114=CARTESIAN_POINT ( 'NONE',  ( -24.95893038578871881, -6.453098109823664608, 47.50000000000011369 ) ) ;
#13126=CARTESIAN_POINT ( 'NONE',  ( -8.779641963837230279, 13.70511383897430058, 48.50000000000012079 ) ) ;
#13127=CARTESIAN_POINT ( 'NONE',  ( -32.80254285330626374, -2.278009980413909563, -48.00000000000012079 ) ) ;
#13139=ADVANCED_FACE ( 'NONE', ( #12538 ), #10227, .T. ) ;
#13144=CARTESIAN_POINT ( 'NONE',  ( -23.02941217286474185, 4.529839663208023559, 48.26891069786830002 ) ) ;
#13157=CARTESIAN_POINT ( 'NONE',  ( -10.80198322015283097, -8.784136766666819085, 47.93908580834070676 ) ) ;
#13158=ORIENTED_EDGE ( 'NONE', *, *, #12183, .F. ) ;
#13163=CARTESIAN_POINT ( 'NONE',  ( -24.12409601409935078, -6.885803942510236197, 58.00000000000012079 ) ) ;
#13165=ORIENTED_EDGE ( 'NONE', *, *, #5916, .T. ) ;
#13167=ORIENTED_EDGE ( 'NONE', *, *, #4717, .T. ) ;
#13175=CARTESIAN_POINT ( 'NONE',  ( -9.391954890838034586, 2.559027098228045638, -47.99579695943414492 ) ) ;
#13182=CARTESIAN_POINT ( 'NONE',  ( -24.78493442214762155, -6.766828585132234508, 47.63220435834860922 ) ) ;
#13184=EDGE_CURVE ( 'NONE', #9911, #7757, #6446, .T. ) ;
#13185=AXIS2_PLACEMENT_3D ( 'NONE', #6627, #11312, #10178 ) ;
#13186=FACE_OUTER_BOUND ( 'NONE', #2897, .T. ) ;
#13191=DIRECTION ( 'NONE',  ( 0.000000000000000000, -0.000000000000000000, -1.000000000000000000 ) ) ;
#13193=EDGE_CURVE ( 'NONE', #505, #10236, #754, .T. ) ;
#13201=AXIS2_PLACEMENT_3D ( 'NONE', #13005, #14229, #6155 ) ;
#13205=VERTEX_POINT ( 'NONE', #9620 ) ;
#13209=FACE_OUTER_BOUND ( 'NONE', #13869, .T. ) ;
#13221=LINE ( 'NONE', #14451, #3276 ) ;
#13223=ADVANCED_FACE ( 'NONE', ( #3682 ), #7074, .F. ) ;
#13224=DIRECTION ( 'NONE',  ( -0.000000000000000000, -0.000000000000000000, 1.000000000000000000 ) ) ;
#13231=FACE_OUTER_BOUND ( 'NONE', #1009, .T. ) ;
#13242=DIRECTION ( 'NONE',  ( 0.000000000000000000, 0.000000000000000000, -1.000000000000000000 ) ) ;
#13246=CARTESIAN_POINT ( 'NONE',  ( -21.66581936427349575, -2.249290599286304371, -50.00000000000012079 ) ) ;
#13250=CARTESIAN_POINT ( 'NONE',  ( -23.87164973098472487, 3.842474614898954144, 48.12459668492483189 ) ) ;
#13258=CARTESIAN_POINT ( 'NONE',  ( -9.456839514482961562, 2.659958822950721835, 57.50000000000012079 ) ) ;
#13263=FACE_OUTER_BOUND ( 'NONE', #5642, .T. ) ;
#13267=CARTESIAN_POINT ( 'NONE',  ( -30.80945343098651890, -5.389243620311580329, 57.50000000000012079 ) ) ;
#13280=ORIENTED_EDGE ( 'NONE', *, *, #1328, .F. ) ;
#13282=CARTESIAN_POINT ( 'NONE',  ( -30.80945343098651890, -5.389243620311580329, -48.50000000000012079 ) ) ;
#13292=ORIENTED_EDGE ( 'NONE', *, *, #11766, .F. ) ;
#13295=ORIENTED_EDGE ( 'NONE', *, *, #11517, .T. ) ;
#13296=CARTESIAN_POINT ( 'NONE',  ( -24.72817752516938228, 2.363221963240404566, 47.50000000000012079 ) ) ;
#13305=DIRECTION ( 'NONE',  ( -0.000000000000000000, -0.000000000000000000, 1.000000000000000000 ) ) ;
#13313=CARTESIAN_POINT ( 'NONE',  ( -23.72465974793126620, 3.743354278179100714, 47.97348817130775700 ) ) ;
#13323=CARTESIAN_POINT ( 'NONE',  ( -16.99999999999998579, -2.249290599286303927, 57.50000000000012079 ) ) ;
#13327=CIRCLE ( 'NONE', #9883, 3.694885682588112896 ) ;
#13337=DIRECTION ( 'NONE',  ( -0.5394184268574414576, 0.8420378618367722057, 0.000000000000000000 ) ) ;
#13338=EDGE_CURVE ( 'NONE', #2898, #13205, #6192, .T. ) ;
#13343=DIRECTION ( 'NONE',  ( 0.000000000000000000, 0.000000000000000000, -1.000000000000000000 ) ) ;
#13355=FACE_OUTER_BOUND ( 'NONE', #4583, .T. ) ;
#13363=EDGE_CURVE ( 'NONE', #10236, #1125, #13892, .T. ) ;
#13366=EDGE_LOOP ( 'NONE', ( #5080, #2353, #5094, #10004 ) ) ;
#13369=ADVANCED_FACE ( 'NONE', ( #13231 ), #12345, .T. ) ;
#13381=ORIENTED_EDGE ( 'NONE', *, *, #2503, .T. ) ;
#13392=CARTESIAN_POINT ( 'NONE',  ( -9.090012166261184134, -7.380334305945262408, -48.00000000000014211 ) ) ;
#13393=CARTESIAN_POINT ( 'NONE',  ( -24.54316048551696028, -7.158540021523408292, 48.50000000000012079 ) ) ;
#13406=DIRECTION ( 'NONE',  ( -0.000000000000000000, -0.000000000000000000, -1.000000000000000000 ) ) ;
#13407=CARTESIAN_POINT ( 'NONE',  ( -24.79038709231510040, -6.757381419356298657, -47.62582736825572738 ) ) ;
#13409=EDGE_CURVE ( 'NONE', #7882, #5809, #7410, .T. ) ;
#13420=AXIS2_PLACEMENT_3D ( 'NONE', #12193, #11043, #9829 ) ;
#13426=CARTESIAN_POINT ( 'NONE',  ( -25.15752072101212278, 2.619472661158555038, -48.00000000000012079 ) ) ;
#13439=AXIS2_PLACEMENT_3D ( 'NONE', #13762, #8072, #6914 ) ;
#13458=AXIS2_PLACEMENT_3D ( 'NONE', #8344, #13033, #2411 ) ;
#13461=ADVANCED_FACE ( 'NONE', ( #3125 ), #5732, .F. ) ;
#13463=ADVANCED_FACE ( 'NONE', ( #730 ), #11076, .T. ) ;
#13466=CARTESIAN_POINT ( 'NONE',  ( -5.040221427466109461, 4.089237592873833371, 58.00000000000012079 ) ) ;
#13484=DIRECTION ( 'NONE',  ( -0.000000000000000000, 0.000000000000000000, 1.000000000000000000 ) ) ;
#13487=DIRECTION ( 'NONE',  ( 1.000000000000000000, 0.000000000000000000, 0.000000000000000000 ) ) ;
#13490=AXIS2_PLACEMENT_3D ( 'NONE', #5964, #8108, #13794 ) ;
#13491=CARTESIAN_POINT ( 'NONE',  ( -5.290523468902621929, 4.522075770548486418, -57.50000000000012079 ) ) ;
#13495=DIRECTION ( 'NONE',  ( -0.5394184268574488961, 0.8420378618367674317, 0.000000000000000000 ) ) ;
#13496=DIRECTION ( 'NONE',  ( -0.000000000000000000, 0.000000000000000000, 1.000000000000000000 ) ) ;
#13500=DIRECTION ( 'NONE',  ( 1.000000000000000000, 0.000000000000000000, 0.000000000000000000 ) ) ;
#13505=LINE ( 'NONE', #14882, #5953 ) ;
#13506=EDGE_CURVE ( 'NONE', #7221, #7147, #1737, .T. ) ;
#13513=VERTEX_POINT ( 'NONE', #12760 ) ;
#13515=CARTESIAN_POINT ( 'NONE',  ( -16.99999999999998579, -2.249290599286303927, 38.00000000000012079 ) ) ;
#13524=FACE_OUTER_BOUND ( 'NONE', #9184, .T. ) ;
#13530=AXIS2_PLACEMENT_3D ( 'NONE', #12827, #6652, #877 ) ;
#13537=CARTESIAN_POINT ( 'NONE',  ( 0.5043391135745837195, 0.8906624217387615339, 48.00000000000012079 ) ) ;
#13541=LINE ( 'NONE', #4149, #10470 ) ;
#13542=AXIS2_PLACEMENT_3D ( 'NONE', #1543, #7235, #8545 ) ;
#13544=FACE_OUTER_BOUND ( 'NONE', #8327, .T. ) ;
#13546=DIRECTION ( 'NONE',  ( -1.000000000000000000, 0.000000000000000000, 0.000000000000000000 ) ) ;
#13548=EDGE_CURVE ( 'NONE', #5507, #8849, #1048, .T. ) ;
#13552=AXIS2_PLACEMENT_3D ( 'NONE', #1304, #10775, #10698 ) ;
#13561=CARTESIAN_POINT ( 'NONE',  ( -1.197457146693716057, -2.220571218158943427, 48.00000000000012079 ) ) ;
#13568=ORIENTED_EDGE ( 'NONE', *, *, #3153, .T. ) ;
#13576=LINE ( 'NONE', #4179, #6458 ) ;
#13578=CARTESIAN_POINT ( 'NONE',  ( 0.000000000000000000, 0.000000000000000000, 58.00000000000012079 ) ) ;
#13587=AXIS2_PLACEMENT_3D ( 'NONE', #10938, #9716, #6170 ) ;
#13589=ADVANCED_FACE ( 'NONE', ( #14285 ), #10350, .F. ) ;
#13603=CARTESIAN_POINT ( 'NONE',  ( -16.99999999999998579, -2.249290599286303927, -38.00000000000012079 ) ) ;
#13604=ORIENTED_EDGE ( 'NONE', *, *, #9123, .T. ) ;
#13606=CARTESIAN_POINT ( 'NONE',  ( -8.499999999999987566, -2.249290599286303927, 38.50000000000012790 ) ) ;
#13607=CARTESIAN_POINT ( 'NONE',  ( -16.99999999999998579, -2.249290599286303927, -47.50000000000012079 ) ) ;
#13608=DIRECTION ( 'NONE',  ( -0.8656763553493062036, -0.5006040828730242698, 0.000000000000000000 ) ) ;
#13609=EDGE_LOOP ( 'NONE', ( #13059, #11387, #11098 ) ) ;
#13612=LINE ( 'NONE', #12305, #4877 ) ;
#13616=DIRECTION ( 'NONE',  ( -0.8420378618367651002, -0.5394184268574528929, -2.807225425332302624E-15 ) ) ;
#13618=CARTESIAN_POINT ( 'NONE',  ( -22.95637227168126770, 4.533106128208347130, -48.03392779025640635 ) ) ;
#13619=DIRECTION ( 'NONE',  ( 1.000000000000000000, 0.000000000000000000, 0.000000000000000000 ) ) ;
#13620=ORIENTED_EDGE ( 'NONE', *, *, #707, .T. ) ;
#13623=CARTESIAN_POINT ( 'NONE',  ( -9.358536206588548012, 2.506280377409947135, 47.89606589046130125 ) ) ;
#13626=CARTESIAN_POINT ( 'NONE',  ( -0.9277479332649583021, -2.641590149077306826, 57.50000000000012079 ) ) ;
#13627=CARTESIAN_POINT ( 'NONE',  ( -5.040221427466046400, 4.089237592873870675, -48.00000000000012079 ) ) ;
#13628=ADVANCED_FACE ( 'NONE', ( #2284 ), #2735, .T. ) ;
#13634=CARTESIAN_POINT ( 'NONE',  ( -16.99999999999998579, -2.249290599286303927, -50.50000000000012079 ) ) ;
#13641=EDGE_CURVE ( 'NONE', #3355, #13079, #5194, .T. ) ;
#13645=CARTESIAN_POINT ( 'NONE',  ( -16.99999999999998579, -2.249290599286303927, -47.31370849898487307 ) ) ;
#13646=VERTEX_POINT ( 'NONE', #10522 ) ;
#13647=LINE ( 'NONE', #944, #8404 ) ;
#13657=CIRCLE ( 'NONE', #397, 0.5000000000000003331 ) ;
#13665=ORIENTED_EDGE ( 'NONE', *, *, #2430, .T. ) ;
#13666=DIRECTION ( 'NONE',  ( 0.000000000000000000, 0.000000000000000000, -1.000000000000000000 ) ) ;
#13670=DIRECTION ( 'NONE',  ( 0.000000000000000000, 0.000000000000000000, -1.000000000000000000 ) ) ;
#13673=EDGE_LOOP ( 'NONE', ( #894, #631, #5531, #2319 ) ) ;
#13681=CARTESIAN_POINT ( 'NONE',  ( -16.99999999999998579, -2.249290599286303927, -57.50000000000012079 ) ) ;
#13683=ORIENTED_EDGE ( 'NONE', *, *, #3414, .T. ) ;
#13694=CIRCLE ( 'NONE', #8042, 4.194885682587998765 ) ;
#13696=CARTESIAN_POINT ( 'NONE',  ( -24.72817752516938228, 2.363221963240404566, -47.50000000000012079 ) ) ;
#13713=CARTESIAN_POINT ( 'NONE',  ( -8.537170960192302260, 2.067018546614597163, 48.00000000000012079 ) ) ;
#13722=CARTESIAN_POINT ( 'NONE',  ( -25.99999999999998934, -2.249290599286303927, 58.00000000000012079 ) ) ;
#13725=EDGE_LOOP ( 'NONE', ( #12787, #636, #4412, #4919 ) ) ;
#13730=EDGE_CURVE ( 'NONE', #11720, #8531, #8720, .T. ) ;
#13733=CYLINDRICAL_SURFACE ( 'NONE', #1395, 0.4999999999999996114 ) ;
#13741=EDGE_CURVE ( 'NONE', #7624, #12008, #12033, .T. ) ;
#13746=VECTOR ( 'NONE', #10319, 1000.000000000000114 ) ;
#13755=EDGE_LOOP ( 'NONE', ( #2730, #13999, #8987, #9853 ) ) ;
#13762=CARTESIAN_POINT ( 'NONE',  ( -16.99999999999998579, -2.249290599286303927, -58.00000000000012079 ) ) ;
#13771=CARTESIAN_POINT ( 'NONE',  ( -16.99999999999998579, -2.249290599286303927, 38.50000000000012790 ) ) ;
#13773=ORIENTED_EDGE ( 'NONE', *, *, #9616, .F. ) ;
#13781=CYLINDRICAL_SURFACE ( 'NONE', #2225, 4.194885682587998765 ) ;
#13783=ORIENTED_EDGE ( 'NONE', *, *, #11242, .T. ) ;
#13794=DIRECTION ( 'NONE',  ( 1.000000000000000000, 0.000000000000000000, 0.000000000000000000 ) ) ;
#13795=FACE_OUTER_BOUND ( 'NONE', #12557, .T. ) ;
#13807=CIRCLE ( 'NONE', #11106, 0.5000000000000004441 ) ;
#13809=ADVANCED_FACE ( 'NONE', ( #13209 ), #7166, .T. ) ;
#13817=CIRCLE ( 'NONE', #4975, 0.4999999999999995559 ) ;
#13822=DIRECTION ( 'NONE',  ( 1.000000000000000000, 0.000000000000000000, 0.000000000000000000 ) ) ;
#13823=ORIENTED_EDGE ( 'NONE', *, *, #14279, .T. ) ;
#13830=EDGE_CURVE ( 'NONE', #8112, #7744, #10862, .T. ) ;
#13832=FACE_BOUND ( 'NONE', #11301, .T. ) ;
#13839=DIRECTION ( 'NONE',  ( 0.000000000000000000, 0.000000000000000000, -1.000000000000000000 ) ) ;
#13862=FACE_OUTER_BOUND ( 'NONE', #9860, .T. ) ;
#13865=VERTEX_POINT ( 'NONE', #12189 ) ;
#13867=CARTESIAN_POINT ( 'NONE',  ( -9.083879796419006780, -7.373836579503426414, -48.00000000000010658 ) ) ;
#13869=EDGE_LOOP ( 'NONE', ( #5043, #7069, #12916, #13885 ) ) ;
#13874=CARTESIAN_POINT ( 'NONE',  ( -16.99999999999998579, -2.249290599286303927, 50.00000000000012079 ) ) ;
#13877=CARTESIAN_POINT ( 'NONE',  ( -32.80254285330629216, -2.278009980413787439, -57.50000000000012079 ) ) ;
#13885=ORIENTED_EDGE ( 'NONE', *, *, #487, .T. ) ;
#13889=EDGE_CURVE ( 'NONE', #9584, #3752, #13647, .T. ) ;
#13891=EDGE_CURVE ( 'NONE', #4611, #6843, #9114, .T. ) ;
#13892=B_SPLINE_CURVE_WITH_KNOTS ( 'NONE', 3,
 ( #13296, #4042, #1742, #444, #6366, #11201, #14384, #12067, #3825, #7457, #9769, #8532 ),
 .UNSPECIFIED., .F., .F.,
 ( 4, 2, 2, 2, 2, 4 ),
 ( 0.000000000000000000, 0.001071381053236910479, 0.002142762106473820958, 0.003214143159710731654, 0.003749833686329185484, 0.004285524212947640181 ),
 .UNSPECIFIED. ) ;
#13894=CARTESIAN_POINT ( 'NONE',  ( -9.456839514482961562, 2.659958822950721835, -57.50000000000012079 ) ) ;
#13897=CARTESIAN_POINT ( 'NONE',  ( -25.21252699837112132, -6.998437922861946880, -48.50000000000012079 ) ) ;
#13898=ORIENTED_EDGE ( 'NONE', *, *, #7417, .F. ) ;
#13905=VECTOR ( 'NONE', #9105, 1000.000000000000000 ) ;
#13920=ORIENTED_EDGE ( 'NONE', *, *, #10106, .T. ) ;
#13925=AXIS2_PLACEMENT_3D ( 'NONE', #3130, #3287, #7679 ) ;
#13937=ORIENTED_EDGE ( 'NONE', *, *, #14807, .F. ) ;
#13945=ORIENTED_EDGE ( 'NONE', *, *, #10360, .T. ) ;
#13947=CARTESIAN_POINT ( 'NONE',  ( -9.657039156986668260, -7.465117833064532249, -47.54128347411995037 ) ) ;
#13949=ORIENTED_EDGE ( 'NONE', *, *, #388, .F. ) ;
#13963=ORIENTED_EDGE ( 'NONE', *, *, #1619, .F. ) ;
#13972=CARTESIAN_POINT ( 'NONE',  ( -12.33418063572647938, -2.249290599286303927, -50.50000000000012079 ) ) ;
#13974=CYLINDRICAL_SURFACE ( 'NONE', #3707, 0.5000000000000000000 ) ;
#13976=DIRECTION ( 'NONE',  ( -0.8656763553492639041, -0.5006040828730973224, -0.000000000000000000 ) ) ;
#13977=DIRECTION ( 'NONE',  ( 1.000000000000000000, 0.000000000000000000, 0.000000000000000000 ) ) ;
#13978=VERTEX_POINT ( 'NONE', #14961 ) ;
#13986=CARTESIAN_POINT ( 'NONE',  ( -28.70947653109703168, -9.020656969121420232, -48.00000000000012079 ) ) ;
#13996=ORIENTED_EDGE ( 'NONE', *, *, #3417, .F. ) ;
#13999=ORIENTED_EDGE ( 'NONE', *, *, #10410, .T. ) ;
#14007=TOROIDAL_SURFACE ( 'NONE', #7369, 9.500000000000001776, 0.5000000000000000000 ) ;
#14009=DIRECTION ( 'NONE',  ( 1.000000000000000000, 0.000000000000000000, 0.000000000000000000 ) ) ;
#14012=CARTESIAN_POINT ( 'NONE',  ( -28.95977857253358323, -8.587818791446789390, 57.50000000000012079 ) ) ;
#14014=DIRECTION ( 'NONE',  ( 1.000000000000000000, 0.000000000000000000, 0.000000000000000000 ) ) ;
#14031=DIRECTION ( 'NONE',  ( 0.000000000000000000, 0.000000000000000000, 1.000000000000000000 ) ) ;
#14041=VERTEX_POINT ( 'NONE', #4730 ) ;
#14049=CARTESIAN_POINT ( 'NONE',  ( -25.22031829551916360, -6.987901215495521789, 48.36903577193041315 ) ) ;
#14059=CARTESIAN_POINT ( 'NONE',  ( -9.875903985900572835, 2.387222743937554181, 57.50000000000012079 ) ) ;
#14061=VERTEX_POINT ( 'NONE', #1187 ) ;
#14071=AXIS2_PLACEMENT_3D ( 'NONE', #11936, #2480, #6029 ) ;
#14076=AXIS2_PLACEMENT_3D ( 'NONE', #7303, #12150, #11060 ) ;
#14083=EDGE_LOOP ( 'NONE', ( #13381, #12963, #12317, #5877 ) ) ;
#14093=DIRECTION ( 'NONE',  ( 0.000000000000000000, 0.000000000000000000, -1.000000000000000000 ) ) ;
#14096=ORIENTED_EDGE ( 'NONE', *, *, #9974, .T. ) ;
#14104=CARTESIAN_POINT ( 'NONE',  ( -10.08688311991301312, -8.022742138608869311, -47.66502101098957667 ) ) ;
#14108=CARTESIAN_POINT ( 'NONE',  ( -9.456839502978525047, 2.659958805273927140, -48.36906329404666849 ) ) ;
#14110=DIRECTION ( 'NONE',  ( -0.000000000000000000, 0.000000000000000000, 1.000000000000000000 ) ) ;
#14112=CARTESIAN_POINT ( 'NONE',  ( -3.285520523749251520, 5.681530634151883419, 48.00000000000012079 ) ) ;
#14116=DIRECTION ( 'NONE',  ( 1.000000000000000000, 0.000000000000000000, 0.000000000000000000 ) ) ;
#14117=ORIENTED_EDGE ( 'NONE', *, *, #3201, .T. ) ;
#14131=CARTESIAN_POINT ( 'NONE',  ( -24.83354747574476207, -6.700581361908810152, 48.23896987259369240 ) ) ;
#14136=ORIENTED_EDGE ( 'NONE', *, *, #8610, .T. ) ;
#14137=ADVANCED_FACE ( 'NONE', ( #4956 ), #8157, .F. ) ;
#14138=DIRECTION ( 'NONE',  ( 0.8381289428352243220, 0.5454721580263371949, 0.000000000000000000 ) ) ;
#14149=FACE_OUTER_BOUND ( 'NONE', #14601, .T. ) ;
#14154=CARTESIAN_POINT ( 'NONE',  ( 0.9298897195970434737, -1.451567674087680837, -48.00000000000012079 ) ) ;
#14165=ORIENTED_EDGE ( 'NONE', *, *, #12183, .T. ) ;
#14168=LINE ( 'NONE', #13246, #10352 ) ;
#14172=CARTESIAN_POINT ( 'NONE',  ( -24.72817752516935741, 2.363221963240438761, 48.00000000000019185 ) ) ;
#14179=VECTOR ( 'NONE', #4432, 1000.000000000000000 ) ;
#14187=CARTESIAN_POINT ( 'NONE',  ( -3.190546569013415379, 0.8906624217387615339, 48.00000000000012079 ) ) ;
#14190=CIRCLE ( 'NONE', #6320, 9.000000000000001776 ) ;
#14202=DIRECTION ( 'NONE',  ( 0.000000000000000000, 0.000000000000000000, -1.000000000000000000 ) ) ;
#14208=CARTESIAN_POINT ( 'NONE',  ( -24.55671735758753726, -7.137878559097176279, 48.23807154671105479 ) ) ;
#14229=DIRECTION ( 'NONE',  ( 0.000000000000000000, 0.000000000000000000, -1.000000000000000000 ) ) ;
#14234=CIRCLE ( 'NONE', #12015, 4.665819364273509073 ) ;
#14242=CIRCLE ( 'NONE', #952, 0.5000000000000004441 ) ;
#14244=CARTESIAN_POINT ( 'NONE',  ( -9.215065577852303846, 2.268247386559545387, -47.63220435834860922 ) ) ;
#14248=CARTESIAN_POINT ( 'NONE',  ( -5.290523468902621929, 4.522075770548486418, 57.50000000000012079 ) ) ;
#14259=CYLINDRICAL_SURFACE ( 'NONE', #14884, 0.5000000000000002220 ) ;
#14274=DIRECTION ( 'NONE',  ( -0.000000000000000000, -0.000000000000000000, 1.000000000000000000 ) ) ;
#14276=CARTESIAN_POINT ( 'NONE',  ( -3.285520523750506516, 5.681530634152946568, -48.50000000000012079 ) ) ;
#14277=DIRECTION ( 'NONE',  ( 1.000000000000000000, 0.000000000000000000, 0.000000000000000000 ) ) ;
#14278=CARTESIAN_POINT ( 'NONE',  ( -25.32021674380207799, -6.838035406461215437, 48.10016682092218332 ) ) ;
#14279=EDGE_CURVE ( 'NONE', #5382, #11723, #13327, .T. ) ;
#14280=TOROIDAL_SURFACE ( 'NONE', #9124, 9.500000000000001776, 0.5000000000000000000 ) ;
#14285=FACE_OUTER_BOUND ( 'NONE', #7825, .T. ) ;
#14290=CIRCLE ( 'NONE', #12812, 0.5000000000000004441 ) ;
#14291=FACE_OUTER_BOUND ( 'NONE', #9228, .T. ) ;
#14292=MANIFOLD_SOLID_BREP ( 'Boss-Extrude17', #4565 ) ;
#14294=CARTESIAN_POINT ( 'NONE',  ( -24.65452791727695114, 3.133494033999976391, 48.02161282446748203 ) ) ;
#14314=ORIENTED_EDGE ( 'NONE', *, *, #2478, .F. ) ;
#14322=CARTESIAN_POINT ( 'NONE',  ( -9.037775043065352065, 2.932694901963889489, -58.00000000000012079 ) ) ;
#14323=CARTESIAN_POINT ( 'NONE',  ( 0.5043391135745837195, 0.8906624217387615339, -48.00000000000012079 ) ) ;
#14324=ORIENTED_EDGE ( 'NONE', *, *, #14807, .T. ) ;
#14326=CARTESIAN_POINT ( 'NONE',  ( -25.15752072101216896, 2.619472661158628313, 48.00000000000012079 ) ) ;
#14333=ORIENTED_EDGE ( 'NONE', *, *, #3153, .F. ) ;
#14335=B_SPLINE_CURVE_WITH_KNOTS ( 'NONE', 3,
 ( #6952, #13392, #5028, #9873, #2850, #2935, #6261, #11084 ),
 .UNSPECIFIED., .F., .F.,
 ( 4, 2, 2, 4 ),
 ( 5.262391672463365372E-17, 0.001077686929059507720, 0.002155373858118960796, 0.004310747716237871285 ),
 .UNSPECIFIED. ) ;
#14339=CARTESIAN_POINT ( 'NONE',  ( -9.166452524254948386, 2.202000163336201410, -48.23896987259320923 ) ) ;
#14341=CYLINDRICAL_SURFACE ( 'NONE', #1055, 0.5000000000000004441 ) ;
#14343=AXIS2_PLACEMENT_3D ( 'NONE', #13681, #13839, #3140 ) ;
#14362=CARTESIAN_POINT ( 'NONE',  ( -21.58505662828840244, 4.908031226326156293, -58.00000000000012079 ) ) ;
#14366=CARTESIAN_POINT ( 'NONE',  ( -25.99999999999998934, -2.249290599286303927, -38.50000000000012790 ) ) ;
#14372=DIRECTION ( 'NONE',  ( 1.000000000000000000, 0.000000000000000000, 0.000000000000000000 ) ) ;
#14378=CARTESIAN_POINT ( 'NONE',  ( -24.12883632398703782, 3.619414784477793301, 48.08465436988272756 ) ) ;
#14381=ORIENTED_EDGE ( 'NONE', *, *, #10744, .T. ) ;
#14384=CARTESIAN_POINT ( 'NONE',  ( -22.94555154978778688, 4.515786682032536525, 48.04486892757390848 ) ) ;
#14385=ORIENTED_EDGE ( 'NONE', *, *, #5771, .F. ) ;
#14387=ORIENTED_EDGE ( 'NONE', *, *, #2478, .T. ) ;
#14390=FACE_OUTER_BOUND ( 'NONE', #9989, .T. ) ;
#14399=CARTESIAN_POINT ( 'NONE',  ( -22.44582411025819368, 4.950411932228481859, 48.32458034485718912 ) ) ;
#14401=ADVANCED_FACE ( 'NONE', ( #4707 ), #12101, .T. ) ;
#14418=ADVANCED_FACE ( 'NONE', ( #9792 ), #5160, .F. ) ;
#14419=AXIS2_PLACEMENT_3D ( 'NONE', #6026, #2558, #6101 ) ;
#14424=CYLINDRICAL_SURFACE ( 'NONE', #646, 0.5000000000000001110 ) ;
#14427=CIRCLE ( 'NONE', #13925, 0.4999999999999994449 ) ;
#14428=AXIS2_PLACEMENT_3D ( 'NONE', #7660, #11187, #1729 ) ;
#14438=CARTESIAN_POINT ( 'NONE',  ( -25.40901433244242114, -6.686340856221296036, 48.00000000000012079 ) ) ;
#14441=AXIS2_PLACEMENT_3D ( 'NONE', #8863, #8711, #12114 ) ;
#14442=VERTEX_POINT ( 'NONE', #3701 ) ;
#14443=CARTESIAN_POINT ( 'NONE',  ( -10.97058782713534164, -9.028420861780718454, 48.26891069786831423 ) ) ;
#14445=DIRECTION ( 'NONE',  ( 1.224646799147353207E-16, -1.000000000000000000, 0.000000000000000000 ) ) ;
#14451=CARTESIAN_POINT ( 'NONE',  ( -12.14523415828296571, -9.827631355817223024, 57.50000000000012079 ) ) ;
#14463=TOROIDAL_SURFACE ( 'NONE', #11753, 8.500000000000000000, 0.5000000000000000000 ) ;
#14465=DIRECTION ( 'NONE',  ( -0.000000000000000000, 0.000000000000000000, 1.000000000000000000 ) ) ;
#14469=DIRECTION ( 'NONE',  ( -0.8656763553492754504, -0.5006040828730772274, -1.896095000761754519E-14 ) ) ;
#14472=EDGE_LOOP ( 'NONE', ( #4996, #7673, #4534, #9498 ) ) ;
#14475=ORIENTED_EDGE ( 'NONE', *, *, #2546, .F. ) ;
#14476=ORIENTED_EDGE ( 'NONE', *, *, #4717, .F. ) ;
#14478=ORIENTED_EDGE ( 'NONE', *, *, #9149, .F. ) ;
#14482=CARTESIAN_POINT ( 'NONE',  ( -33.07225206673494711, -1.856991049495498425, 48.50000000000012079 ) ) ;
#14488=AXIS2_PLACEMENT_3D ( 'NONE', #687, #9004, #1995 ) ;
#14489=VECTOR ( 'NONE', #11543, 1000.000000000000000 ) ;
#14494=DIRECTION ( 'NONE',  ( 0.8656763553493062036, 0.5006040828730242698, 0.000000000000000000 ) ) ;
#14503=CARTESIAN_POINT ( 'NONE',  ( -24.54316049702162772, -7.158540003846257882, -48.36906329404664007 ) ) ;
#14508=CIRCLE ( 'NONE', #10081, 9.000000000000001776 ) ;
#14509=ORIENTED_EDGE ( 'NONE', *, *, #9276, .F. ) ;
#14513=VERTEX_POINT ( 'NONE', #3844 ) ;
#14521=ORIENTED_EDGE ( 'NONE', *, *, #10069, .T. ) ;
#14526=CIRCLE ( 'NONE', #7889, 0.4999999999999997224 ) ;
#14527=ORIENTED_EDGE ( 'NONE', *, *, #6175, .F. ) ;
#14531=DIRECTION ( 'NONE',  ( 1.000000000000000000, 0.000000000000000000, 0.000000000000000000 ) ) ;
#14543=( GEOMETRIC_REPRESENTATION_CONTEXT ( 3 ) GLOBAL_UNCERTAINTY_ASSIGNED_CONTEXT ( ( #13056 ) ) GLOBAL_UNIT_ASSIGNED_CONTEXT ( ( #10177, #4309, #2006 ) ) REPRESENTATION_CONTEXT ( 'NONE', 'WORKASPACE' ) );
#14545=CIRCLE ( 'NONE', #1273, 9.000000000000001776 ) ;
#14551=CARTESIAN_POINT ( 'NONE',  ( -11.86108202630535224, -9.639858853941328576, -48.38337049880509255 ) ) ;
#14560=AXIS2_PLACEMENT_3D ( 'NONE', #4674, #9297, #1122 ) ;
#14561=CARTESIAN_POINT ( 'NONE',  ( -9.456839514482959785, 2.659958822950722279, 48.50000000000011369 ) ) ;
#14565=AXIS2_PLACEMENT_3D ( 'NONE', #10276, #14966, #12655 ) ;
#14572=LINE ( 'NONE', #11107, #990 ) ;
#14584=DIRECTION ( 'NONE',  ( 1.000000000000000000, 0.000000000000000000, 0.000000000000000000 ) ) ;
#14590=ORIENTED_EDGE ( 'NONE', *, *, #4616, .F. ) ;
#14592=CARTESIAN_POINT ( 'NONE',  ( -21.16581936427349575, -2.249290599286303483, 50.50000000000012079 ) ) ;
#14593=EDGE_LOOP ( 'NONE', ( #4550, #14381, #2822, #6956 ) ) ;
#14600=CARTESIAN_POINT ( 'NONE',  ( -9.271822474830662131, -6.861803161813125662, 47.50000000000012079 ) ) ;
#14601=EDGE_LOOP ( 'NONE', ( #1979, #6353, #13665, #9605, #9487, #3475, #2387, #10192, #375, #10359 ) ) ;
#14605=DIRECTION ( 'NONE',  ( -0.000000000000000000, 0.000000000000000000, 1.000000000000000000 ) ) ;
#14606=DIRECTION ( 'NONE',  ( -0.5394184268574523378, 0.8420378618367652113, 0.000000000000000000 ) ) ;
#14609=ORIENTED_EDGE ( 'NONE', *, *, #15218, .T. ) ;
#14610=ORIENTED_EDGE ( 'NONE', *, *, #6974, .F. ) ;
#14618=CARTESIAN_POINT ( 'NONE',  ( -10.80198322015283097, -8.784136766666819085, -47.93908580834070676 ) ) ;
#14619=ORIENTED_EDGE ( 'NONE', *, *, #3030, .T. ) ;
#14622=CARTESIAN_POINT ( 'NONE',  ( -25.49999999999998934, -2.249290599286304815, -38.00000000000012079 ) ) ;
#14626=CARTESIAN_POINT ( 'NONE',  ( -9.391954890838034586, 2.559027098228045638, 47.99579695943414492 ) ) ;
#14627=EDGE_CURVE ( 'NONE', #7613, #2221, #80, .T. ) ;
#14635=FACE_OUTER_BOUND ( 'NONE', #11537, .T. ) ;
#14637=CARTESIAN_POINT ( 'NONE',  ( -24.54316048551696028, -7.158540021523408292, -57.50000000000012079 ) ) ;
#14638=DIRECTION ( 'NONE',  ( -0.000000000000000000, 0.000000000000000000, 1.000000000000000000 ) ) ;
#14642=EDGE_CURVE ( 'NONE', #9111, #355, #6948, .T. ) ;
#14645=CARTESIAN_POINT ( 'NONE',  ( -21.85476584171713199, 5.329050157244540564, 57.50000000000012079 ) ) ;
#14650=CARTESIAN_POINT ( 'NONE',  ( -1.197457146693715613, -2.220571218158943871, 48.50000000000012079 ) ) ;
#14652=CIRCLE ( 'NONE', #2383, 9.000000000000001776 ) ;
#14653=AXIS2_PLACEMENT_3D ( 'NONE', #13578, #14728, #13500 ) ;
#14670=DIRECTION ( 'NONE',  ( 1.000000000000000000, 1.782910239198384762E-15, 0.000000000000000000 ) ) ;
#14676=FACE_OUTER_BOUND ( 'NONE', #10694, .T. ) ;
#14677=ORIENTED_EDGE ( 'NONE', *, *, #9616, .T. ) ;
#14683=CIRCLE ( 'NONE', #12467, 4.665819364273509073 ) ;
#14698=AXIS2_PLACEMENT_3D ( 'NONE', #1197, #12978, #14277 ) ;
#14699=CARTESIAN_POINT ( 'NONE',  ( -8.655068852960594583, 2.300722221922764543, -48.05421924268924272 ) ) ;
#14705=VERTEX_POINT ( 'NONE', #4900 ) ;
#14706=FACE_OUTER_BOUND ( 'NONE', #231, .T. ) ;
#14707=DIRECTION ( 'NONE',  ( -0.000000000000000000, 0.000000000000000000, 1.000000000000000000 ) ) ;
#14712=ORIENTED_EDGE ( 'NONE', *, *, #10035, .F. ) ;
#14716=ADVANCED_FACE ( 'NONE', ( #12351 ), #6282, .T. ) ;
#14727=CARTESIAN_POINT ( 'NONE',  ( -9.871163676013017252, -8.117995983050501962, 48.08465436988272046 ) ) ;
#14728=DIRECTION ( 'NONE',  ( -0.000000000000000000, 0.000000000000000000, 1.000000000000000000 ) ) ;
#14729=CIRCLE ( 'NONE', #3438, 4.000000000000000000 ) ;
#14733=CARTESIAN_POINT ( 'NONE',  ( -12.33418063572647938, -2.249290599286303927, 57.50000000000012079 ) ) ;
#14736=LINE ( 'NONE', #11195, #14927 ) ;
#14745=CARTESIAN_POINT ( 'NONE',  ( -25.21252699837112132, -6.998437922861947769, -57.50000000000012079 ) ) ;
#14747=DIRECTION ( 'NONE',  ( -0.000000000000000000, -0.000000000000000000, 1.000000000000000000 ) ) ;
#14756=ORIENTED_EDGE ( 'NONE', *, *, #2725, .T. ) ;
#14770=CARTESIAN_POINT ( 'NONE',  ( -9.271822474830662131, -6.861803161813125662, -47.50000000000012079 ) ) ;
#14771=AXIS2_PLACEMENT_3D ( 'NONE', #9995, #9856, #7469 ) ;
#14773=DIRECTION ( 'NONE',  ( -0.000000000000000000, 0.000000000000000000, 1.000000000000000000 ) ) ;
#14775=DIRECTION ( 'NONE',  ( 1.000000000000000000, -8.673617379884027583E-15, 0.000000000000000000 ) ) ;
#14779=ORIENTED_EDGE ( 'NONE', *, *, #6974, .T. ) ;
#14784=ORIENTED_EDGE ( 'NONE', *, *, #4423, .F. ) ;
#14786=CARTESIAN_POINT ( 'NONE',  ( -9.456839514482961562, 2.659958822950722723, -58.00000000000012079 ) ) ;
#14789=VERTEX_POINT ( 'NONE', #12048 ) ;
#14795=CARTESIAN_POINT ( 'NONE',  ( -24.99086469133269617, -6.390485686409522081, -48.00342231809331395 ) ) ;
#14797=DIRECTION ( 'NONE',  ( -0.000000000000000000, -0.000000000000000000, 1.000000000000000000 ) ) ;
#14798=AXIS2_PLACEMENT_3D ( 'NONE', #8880, #872, #9119 ) ;
#14807=EDGE_CURVE ( 'NONE', #15152, #12155, #9457, .T. ) ;
#14808=AXIS2_PLACEMENT_3D ( 'NONE', #9734, #1564, #1630 ) ;
#14814=CIRCLE ( 'NONE', #2539, 9.000000000000001776 ) ;
#14816=CARTESIAN_POINT ( 'NONE',  ( -23.85820543185402798, 3.853856159079054322, -48.12676452506695313 ) ) ;
#14817=AXIS2_PLACEMENT_3D ( 'NONE', #11776, #3839, #3918 ) ;
#14823=DIRECTION ( 'NONE',  ( 0.8420378618367675427, 0.5394184268574490071, -0.000000000000000000 ) ) ;
#14828=DIRECTION ( 'NONE',  ( 1.000000000000000000, 0.000000000000000000, 0.000000000000000000 ) ) ;
#14846=CARTESIAN_POINT ( 'NONE',  ( -23.95855436784179560, 3.468451880982295954, -47.93156476714377590 ) ) ;
#14865=CARTESIAN_POINT ( 'NONE',  ( -8.842479278987921631, -7.118053859731281463, 47.50000000000012079 ) ) ;
#14875=EDGE_LOOP ( 'NONE', ( #11418, #3606, #8734, #7617 ) ) ;
#14877=DIRECTION ( 'NONE',  ( 1.000000000000000000, 0.000000000000000000, 0.000000000000000000 ) ) ;
#14882=CARTESIAN_POINT ( 'NONE',  ( -32.80254285330622110, -2.278009980413881141, 58.00000000000012079 ) ) ;
#14884=AXIS2_PLACEMENT_3D ( 'NONE', #7248, #5884, #8265 ) ;
#14901=DIRECTION ( 'NONE',  ( 0.5006040828730246028, -0.8656763553493059815, 0.000000000000000000 ) ) ;
#14906=DIRECTION ( 'NONE',  ( 0.000000000000000000, 0.000000000000000000, -1.000000000000000000 ) ) ;
#14908=CARTESIAN_POINT ( 'NONE',  ( -11.57001547143821085, -9.459140135624386048, 48.26605223432068925 ) ) ;
#14911=CARTESIAN_POINT ( 'NONE',  ( -24.54316048551696028, -7.158540021523408292, -58.00000000000012079 ) ) ;
#14920=CIRCLE ( 'NONE', #5333, 0.4999999999999999445 ) ;
#14922=CARTESIAN_POINT ( 'NONE',  ( -22.44582411025819368, 4.950411932228481859, -48.32458034485718912 ) ) ;
#14925=DIRECTION ( 'NONE',  ( -0.8420378618367728718, -0.5394184268574404584, -0.000000000000000000 ) ) ;
#14927=VECTOR ( 'NONE', #7449, 1000.000000000000000 ) ;
#14939=CARTESIAN_POINT ( 'NONE',  ( -8.779641963837230279, 13.70511383897430058, -48.50000000000012079 ) ) ;
#14951=CARTESIAN_POINT ( 'NONE',  ( -9.198099351547387670, 2.262399358110477543, -48.50000000000012079 ) ) ;
#14955=FACE_OUTER_BOUND ( 'NONE', #6009, .T. ) ;
#14956=EDGE_CURVE ( 'NONE', #10712, #6376, #12859, .T. ) ;
#14959=ORIENTED_EDGE ( 'NONE', *, *, #6175, .T. ) ;
#14961=CARTESIAN_POINT ( 'NONE',  ( -8.982583014919022446, 1.839844381040865118, -47.50000000000012079 ) ) ;
#14963=EDGE_CURVE ( 'NONE', #4994, #3246, #13576, .T. ) ;
#14966=DIRECTION ( 'NONE',  ( -0.000000000000000000, 0.000000000000000000, 1.000000000000000000 ) ) ;
#14979=DIRECTION ( 'NONE',  ( 0.000000000000000000, 0.000000000000000000, -1.000000000000000000 ) ) ;
#14985=DIRECTION ( 'NONE',  ( 0.000000000000000000, -0.000000000000000000, -1.000000000000000000 ) ) ;
#15005=ADVANCED_FACE ( 'NONE', ( #5579 ), #1028, .F. ) ;
#15007=DIRECTION ( 'NONE',  ( 0.8908241094534407045, 0.4543483311474627029, 0.000000000000000000 ) ) ;
#15013=FACE_BOUND ( 'NONE', #10559, .T. ) ;
#15020=VERTEX_POINT ( 'NONE', #8039 ) ;
#15021=DIRECTION ( 'NONE',  ( 1.000000000000000000, 0.000000000000000000, 0.000000000000000000 ) ) ;
#15027=CARTESIAN_POINT ( 'NONE',  ( -9.875903985900572835, 2.387222743937554181, -57.50000000000012079 ) ) ;
#15034=PLANE ( 'NONE',  #12770 ) ;
#15041=CARTESIAN_POINT ( 'NONE',  ( -3.190546569013415379, 0.8906624217387615339, -48.00000000000012079 ) ) ;
#15049=ADVANCED_FACE ( 'NONE', ( #1259 ), #10729, .T. ) ;
#15057=VECTOR ( 'NONE', #1244, 1000.000000000000000 ) ;
#15078=CARTESIAN_POINT ( 'NONE',  ( -11.04362772831848716, -9.031687326780717839, 48.03392779025379156 ) ) ;
#15079=ORIENTED_EDGE ( 'NONE', *, *, #901, .T. ) ;
#15086=ORIENTED_EDGE ( 'NONE', *, *, #3917, .T. ) ;
#15087=CARTESIAN_POINT ( 'NONE',  ( -9.271822474830662131, -6.861803161813125662, 47.50000000000012079 ) ) ;
#15108=DIRECTION ( 'NONE',  ( 1.000000000000000000, 0.000000000000000000, 0.000000000000000000 ) ) ;
#15110=FACE_OUTER_BOUND ( 'NONE', #12714, .T. ) ;
#15123=DIRECTION ( 'NONE',  ( 0.8656763553492640151, 0.5006040828730974335, 0.000000000000000000 ) ) ;
#15130=DIRECTION ( 'NONE',  ( 1.000000000000000000, 0.000000000000000000, 0.000000000000000000 ) ) ;
#15134=ORIENTED_EDGE ( 'NONE', *, *, #13548, .F. ) ;
#15139=AXIS2_PLACEMENT_3D ( 'NONE', #12643, #4316, #11397 ) ;
#15146=CARTESIAN_POINT ( 'NONE',  ( -10.12835026901530178, -8.341055813471566438, 48.12459668492476084 ) ) ;
#15149=CARTESIAN_POINT ( 'NONE',  ( -25.21252699837112132, -6.998437922861946880, 48.50000000000012079 ) ) ;
#15151=CARTESIAN_POINT ( 'NONE',  ( -8.787473001628837821, 2.499856724289235554, 57.50000000000012079 ) ) ;
#15152=VERTEX_POINT ( 'NONE', #11728 ) ;
#15158=AXIS2_PLACEMENT_3D ( 'NONE', #8743, #5070, #9776 ) ;
#15159=DIRECTION ( 'NONE',  ( 1.000000000000000000, 0.000000000000000000, 0.000000000000000000 ) ) ;
#15166=VECTOR ( 'NONE', #4372, 1000.000000000000000 ) ;
#15176=( NAMED_UNIT ( * ) SI_UNIT ( $, .STERADIAN. ) SOLID_ANGLE_UNIT ( ) );
#15185=EDGE_CURVE ( 'NONE', #12155, #5046, #9273, .T. ) ;
#15190=DIRECTION ( 'NONE',  ( 1.000000000000000000, 0.000000000000000000, 0.000000000000000000 ) ) ;
#15201=ADVANCED_FACE ( 'NONE', ( #267 ), #14424, .T. ) ;
#15205=CARTESIAN_POINT ( 'NONE',  ( -24.96222495693456978, -7.431276100536581275, 58.00000000000012079 ) ) ;
#15207=ORIENTED_EDGE ( 'NONE', *, *, #5554, .F. ) ;
#15209=UNCERTAINTY_MEASURE_WITH_UNIT (LENGTH_MEASURE( 1.000000000000000082E-05 ), #9484, 'distance_accuracy_value', 'NONE');
#15211=DIRECTION ( 'NONE',  ( 1.000000000000000000, 0.000000000000000000, 0.000000000000000000 ) ) ;
#15216=( BOUNDED_SURFACE ( )  B_SPLINE_SURFACE ( 3, 2, ( 
 ( #11808, #8507, #127 ),
 ( #9512, #13051, #9596 ),
 ( #14208, #9358, #14049 ),
 ( #12906, #14131, #6050 ),
 ( #7041, #8284, #3511 ),
 ( #2582, #3662, #14278 ),
 ( #48, #7125, #10587 ),
 ( #1421, #274, #12979 ),
 ( #10737, #8362, #1268 ),
 ( #5981, #198, #1198 ) ),
 .UNSPECIFIED., .F., .F., .F. ) 
 B_SPLINE_SURFACE_WITH_KNOTS ( ( 4, 2, 2, 2, 4 ),
 ( 3, 3 ),
 ( 0.0006711510808134562266, 0.001062132081067026709, 0.001453113081320597409, 0.001844094081574168108, 0.002235075081827738591 ),
 ( 0.000000000000000000, 1.000000000000000000 ),
 .UNSPECIFIED. ) 
 GEOMETRIC_REPRESENTATION_ITEM ( )  RATIONAL_B_SPLINE_SURFACE ( (
 ( 1.000000000000000000, 0.7254762501099963901, 1.000000000000000000),
 ( 1.000000000000000000, 0.7255094664176422459, 1.000000000000000000),
 ( 1.000000000000000000, 0.7239949553644952074, 1.000000000000000000),
 ( 1.000000000000000000, 0.7190573720639429345, 1.000000000000000000),
 ( 1.000000000000000000, 0.7156412189950915881, 1.000000000000000000),
 ( 1.000000000000000000, 0.7094102539594338008, 1.000000000000000000),
 ( 1.000000000000000000, 0.7066203625162998936, 1.000000000000000000),
 ( 1.000000000000000000, 0.7042417591947802702, 1.000000000000000000),
 ( 1.000000000000000000, 0.7046402682201203804, 1.000000000000000000),
 ( 1.000000000000000000, 0.7071067811865500152, 1.000000000000000000) ) ) 
 REPRESENTATION_ITEM ( '' )  SURFACE ( )  );
#15218=EDGE_CURVE ( 'NONE', #14513, #11720, #10503, .T. ) ;
#15219=DIRECTION ( 'NONE',  ( -0.8656763553493062036, -0.5006040828730242698, -0.000000000000000000 ) ) ;
#15222=DIRECTION ( 'NONE',  ( 0.000000000000000000, -0.000000000000000000, -1.000000000000000000 ) ) ;
#15259=COLOUR_RGB('Grey',0.48,0.52,0.57);
#15260=FILL_AREA_STYLE_COLOUR('',#15259);
#15261=FILL_AREA_STYLE('',(#15260));
#15262=SURFACE_STYLE_FILL_AREA(#15261);
#15263=SURFACE_SIDE_STYLE('',(#15262));
#15264=SURFACE_STYLE_USAGE(.BOTH.,#15263);
#15265=PRESENTATION_STYLE_ASSIGNMENT((#15264));
ENDSEC;
END-ISO-10303-21;
